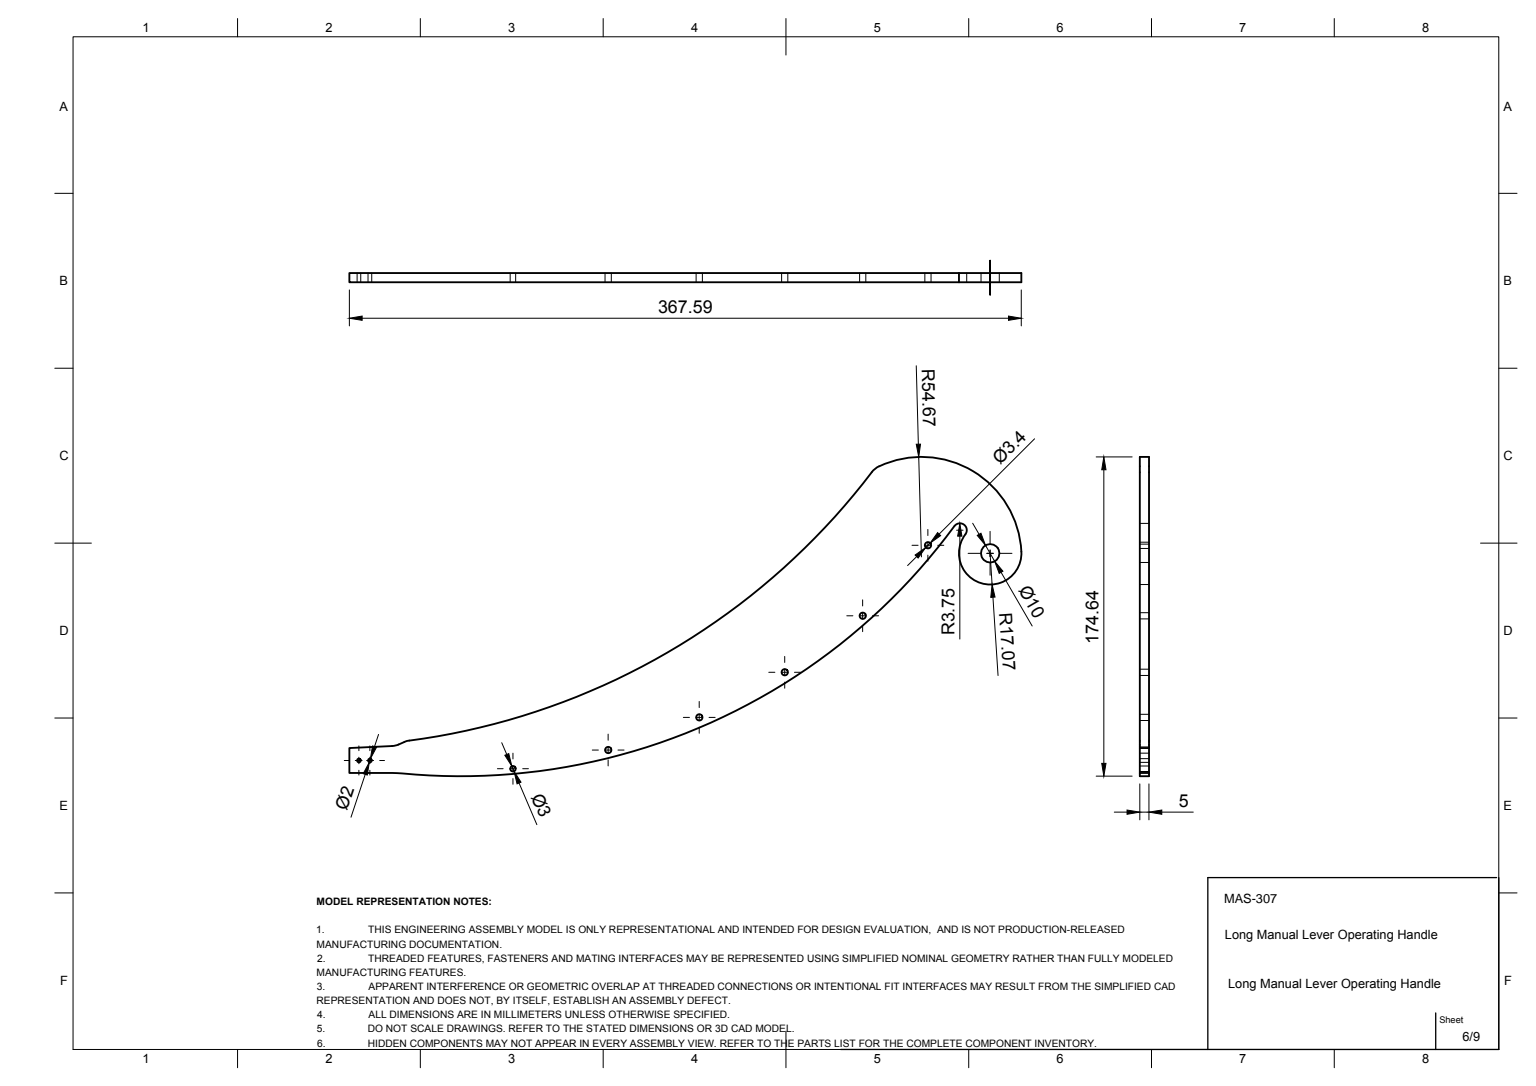
ISO-10303-21;
HEADER;
FILE_DESCRIPTION (('STEP AP214'),
    '1' );
FILE_NAME ('Long Manual Lever Operating Handle.step',
    '2026-10-06T07:34:29',
    ( '' ),
    ( '' ),
    'SwSTEP 2.0',
    'SolidWorks 2025',
    '' );
FILE_SCHEMA (( 'AUTOMOTIVE_DESIGN' ));
ENDSEC;

DATA;
#26=LINE ( 'NONE', #1296, #2230 ) ;
#32=ORIENTED_EDGE ( 'NONE', *, *, #11983, .F. ) ;
#34=DIRECTION ( 'NONE',  ( -0.000000000000000000, -0.000000000000000000, 1.000000000000000000 ) ) ;
#57=DIRECTION ( 'NONE',  ( 1.000000000000000000, 0.000000000000000000, 0.000000000000000000 ) ) ;
#79=ORIENTED_EDGE ( 'NONE', *, *, #3059, .T. ) ;
#100=DIRECTION ( 'NONE',  ( -1.000000000000000000, 0.000000000000000000, 0.000000000000000000 ) ) ;
#106=CYLINDRICAL_SURFACE ( 'NONE', #2526, 3.752352628381527833 ) ;
#107=LINE ( 'NONE', #4949, #8591 ) ;
#149=ORIENTED_EDGE ( 'NONE', *, *, #15360, .T. ) ;
#179=DIRECTION ( 'NONE',  ( 0.000000000000000000, 0.000000000000000000, 1.000000000000000000 ) ) ;
#192=ORIENTED_EDGE ( 'NONE', *, *, #11037, .F. ) ;
#214=VECTOR ( 'NONE', #12787, 1000.000000000000227 ) ;
#215=ORIENTED_EDGE ( 'NONE', *, *, #12661, .T. ) ;
#230=EDGE_LOOP ( 'NONE', ( #7966, #6489 ) ) ;
#255=DIRECTION ( 'NONE',  ( -0.000000000000000000, -0.000000000000000000, 1.000000000000000000 ) ) ;
#261=VECTOR ( 'NONE', #6975, 1000.000000000000000 ) ;
#284=CARTESIAN_POINT ( 'NONE',  ( 71.96535645333923981, 38.79159067395544014, 0.000000000000000000 ) ) ;
#289=AXIS2_PLACEMENT_3D ( 'NONE', #7420, #5036, #8676 ) ;
#295=VERTEX_POINT ( 'NONE', #2676 ) ;
#307=( NAMED_UNIT ( * ) SI_UNIT ( $, .STERADIAN. ) SOLID_ANGLE_UNIT ( ) );
#320=AXIS2_PLACEMENT_3D ( 'NONE', #10803, #2269, #8291 ) ;
#343=MECHANICAL_DESIGN_GEOMETRIC_PRESENTATION_REPRESENTATION('',(#14469),#13976);
#344=CARTESIAN_POINT ( 'NONE',  ( 70.26535645333922275, 38.79159067395544014, 5.000000000000000000 ) ) ;
#362=EDGE_CURVE ( 'NONE', #3997, #6369, #2486, .T. ) ;
#380=EDGE_CURVE ( 'NONE', #4418, #13651, #9757, .T. ) ;
#392=EDGE_CURVE ( 'NONE', #873, #13090, #3748, .T. ) ;
#401=EDGE_CURVE ( 'NONE', #462, #12631, #776, .T. ) ;
#437=CARTESIAN_POINT ( 'NONE',  ( -157.8787660911425803, 118.6941998492684149, 0.000000000000000000 ) ) ;
#462=VERTEX_POINT ( 'NONE', #13132 ) ;
#479=DIRECTION ( 'NONE',  ( 1.000000000000000000, 0.000000000000000000, 0.000000000000000000 ) ) ;
#518=EDGE_CURVE ( 'NONE', #13949, #12631, #4054, .T. ) ;
#523=AXIS2_PLACEMENT_3D ( 'NONE', #7628, #7709, #8968 ) ;
#535=ADVANCED_FACE ( 'NONE', ( #6521 ), #1971, .F. ) ;
#539=DIRECTION ( 'NONE',  ( 0.000000000000000000, 0.000000000000000000, 1.000000000000000000 ) ) ;
#545=CARTESIAN_POINT ( 'NONE',  ( -83.77455057502459113, 65.19100426474074084, 0.000000000000000000 ) ) ;
#548=DIRECTION ( 'NONE',  ( -1.000000000000000000, 0.000000000000000000, 0.000000000000000000 ) ) ;
#555=VERTEX_POINT ( 'NONE', #2885 ) ;
#565=VECTOR ( 'NONE', #10580, 1000.000000000000000 ) ;
#595=CARTESIAN_POINT ( 'NONE',  ( -164.5262273476079713, 106.7842295329138835, 5.000000000000000000 ) ) ;
#603=DIRECTION ( 'NONE',  ( 1.000000000000000000, 0.000000000000000000, 0.000000000000000000 ) ) ;
#617=LINE ( 'NONE', #4250, #8359 ) ;
#631=ORIENTED_EDGE ( 'NONE', *, *, #14587, .T. ) ;
#653=AXIS2_PLACEMENT_3D ( 'NONE', #7411, #179, #5028 ) ;
#667=ORIENTED_EDGE ( 'NONE', *, *, #9159, .T. ) ;
#673=CARTESIAN_POINT ( 'NONE',  ( -130.9946291778373961, 96.97121815129470690, 5.000000000000000000 ) ) ;
#678=AXIS2_PLACEMENT_3D ( 'NONE', #4721, #11915, #10972 ) ;
#679=FACE_BOUND ( 'NONE', #3096, .T. ) ;
#680=DIRECTION ( 'NONE',  ( 1.000000000000000000, 0.000000000000000000, 0.000000000000000000 ) ) ;
#681=EDGE_CURVE ( 'NONE', #5691, #12864, #13249, .T. ) ;
#697=ORIENTED_EDGE ( 'NONE', *, *, #1397, .T. ) ;
#751=CARTESIAN_POINT ( 'NONE',  ( 122.5806775638430253, 45.00321902537314145, 10.00000000000000178 ) ) ;
#760=CIRCLE ( 'NONE', #10878, 17.06579782980005433 ) ;
#768=CYLINDRICAL_SURFACE ( 'NONE', #9832, 1.699999999999993072 ) ;
#776=CIRCLE ( 'NONE', #15400, 5.000000000000004441 ) ;
#817=AXIS2_PLACEMENT_3D ( 'NONE', #1888, #15144, #9176 ) ;
#822=EDGE_CURVE ( 'NONE', #13988, #1469, #4075, .T. ) ;
#825=DIRECTION ( 'NONE',  ( -0.000000000000000000, -0.000000000000000000, -1.000000000000000000 ) ) ;
#839=EDGE_CURVE ( 'NONE', #6369, #8350, #8141, .T. ) ;
#844=FACE_BOUND ( 'NONE', #3836, .T. ) ;
#846=ORIENTED_EDGE ( 'NONE', *, *, #12928, .T. ) ;
#860=AXIS2_PLACEMENT_3D ( 'NONE', #12437, #4145, #5109 ) ;
#873=VERTEX_POINT ( 'NONE', #10108 ) ;
#876=CARTESIAN_POINT ( 'NONE',  ( 200.1062858801516597, 40.86394065090267702, 5.000000000000000000 ) ) ;
#895=EDGE_CURVE ( 'NONE', #11510, #13090, #8296, .T. ) ;
#902=DIRECTION ( 'NONE',  ( 0.000000000000000000, 0.000000000000000000, 1.000000000000000000 ) ) ;
#913=CARTESIAN_POINT ( 'NONE',  ( -150.4086188282879277, 107.2728346664360259, 0.000000000000000000 ) ) ;
#916=EDGE_CURVE ( 'NONE', #14981, #2732, #12150, .T. ) ;
#920=CYLINDRICAL_SURFACE ( 'NONE', #10681, 1.500000000000001332 ) ;
#955=ORIENTED_EDGE ( 'NONE', *, *, #7157, .T. ) ;
#963=ORIENTED_EDGE ( 'NONE', *, *, #5376, .T. ) ;
#970=CIRCLE ( 'NONE', #11577, 335.5619230110239641 ) ;
#1018=EDGE_LOOP ( 'NONE', ( #2531, #11475, #6093, #963 ) ) ;
#1037=CARTESIAN_POINT ( 'NONE',  ( -156.6477983077465410, 110.1970436846185066, -5.000000000000000000 ) ) ;
#1040=VECTOR ( 'NONE', #1882, 1000.000000000000227 ) ;
#1046=CARTESIAN_POINT ( 'NONE',  ( -135.3034657297974093, 107.4444500778096483, 5.000000000000000000 ) ) ;
#1059=ADVANCED_FACE ( 'NONE', ( #12139 ), #2593, .T. ) ;
#1071=VERTEX_POINT ( 'NONE', #6301 ) ;
#1092=DIRECTION ( 'NONE',  ( -0.000000000000000000, -0.000000000000000000, -1.000000000000000000 ) ) ;
#1121=DIRECTION ( 'NONE',  ( 1.000000000000000000, 0.000000000000000000, 0.000000000000000000 ) ) ;
#1126=VERTEX_POINT ( 'NONE', #4961 ) ;
#1152=DIRECTION ( 'NONE',  ( 1.000000000000000000, 0.000000000000000000, 0.000000000000000000 ) ) ;
#1153=DIRECTION ( 'NONE',  ( 0.000000000000000000, 0.000000000000000000, 1.000000000000000000 ) ) ;
#1163=EDGE_CURVE ( 'NONE', #4062, #3314, #3306, .T. ) ;
#1174=ORIENTED_EDGE ( 'NONE', *, *, #12928, .F. ) ;
#1197=ORIENTED_EDGE ( 'NONE', *, *, #13835, .T. ) ;
#1201=ADVANCED_FACE ( 'NONE', ( #14881 ), #9062, .F. ) ;
#1213=DIRECTION ( 'NONE',  ( 0.000000000000000000, 0.000000000000000000, 1.000000000000000000 ) ) ;
#1223=DIRECTION ( 'NONE',  ( 1.000000000000000000, 0.000000000000000000, 0.000000000000000000 ) ) ;
#1247=CIRCLE ( 'NONE', #3275, 1.000000000000000888 ) ;
#1252=AXIS2_PLACEMENT_3D ( 'NONE', #10138, #10216, #6512 ) ;
#1269=VERTEX_POINT ( 'NONE', #11422 ) ;
#1270=ORIENTED_EDGE ( 'NONE', *, *, #2769, .F. ) ;
#1296=CARTESIAN_POINT ( 'NONE',  ( -157.6477983077465694, 110.1970436846185066, -5.000000000000000000 ) ) ;
#1303=AXIS2_PLACEMENT_3D ( 'NONE', #9004, #12617, #1876 ) ;
#1312=FACE_OUTER_BOUND ( 'NONE', #2942, .T. ) ;
#1321=CYLINDRICAL_SURFACE ( 'NONE', #6253, 1.700000000000007061 ) ;
#1336=ORIENTED_EDGE ( 'NONE', *, *, #8208, .T. ) ;
#1388=EDGE_LOOP ( 'NONE', ( #7148, #8695 ) ) ;
#1397=EDGE_CURVE ( 'NONE', #14981, #13397, #2338, .T. ) ;
#1447=VERTEX_POINT ( 'NONE', #2261 ) ;
#1454=DIRECTION ( 'NONE',  ( 0.000000000000000000, 0.000000000000000000, 1.000000000000000000 ) ) ;
#1459=VECTOR ( 'NONE', #9027, 1000.000000000000000 ) ;
#1469=VERTEX_POINT ( 'NONE', #3451 ) ;
#1497=CIRCLE ( 'NONE', #10338, 9.999999999999994671 ) ;
#1508=EDGE_CURVE ( 'NONE', #11510, #12123, #1497, .T. ) ;
#1523=ADVANCED_FACE ( 'NONE', ( #15584 ), #7177, .F. ) ;
#1563=DIRECTION ( 'NONE',  ( -0.000000000000000000, -0.000000000000000000, 1.000000000000000000 ) ) ;
#1584=VERTEX_POINT ( 'NONE', #7772 ) ;
#1593=ORIENTED_EDGE ( 'NONE', *, *, #7358, .F. ) ;
#1598=DIRECTION ( 'NONE',  ( 0.9951762285753402715, -0.09810338464376282264, 0.000000000000000000 ) ) ;
#1625=EDGE_CURVE ( 'NONE', #11700, #462, #12561, .T. ) ;
#1644=EDGE_LOOP ( 'NONE', ( #4661, #10401 ) ) ;
#1648=ADVANCED_FACE ( 'NONE', ( #13749 ), #4122, .F. ) ;
#1674=CARTESIAN_POINT ( 'NONE',  ( 170.2911098586863545, 111.9959133412127272, 5.000000000000000000 ) ) ;
#1678=FACE_OUTER_BOUND ( 'NONE', #14769, .T. ) ;
#1681=CARTESIAN_POINT ( 'NONE',  ( -34.79899788034579444, 48.72489408690345414, 10.00000000000000178 ) ) ;
#1694=ADVANCED_FACE ( 'NONE', ( #1678 ), #5396, .T. ) ;
#1717=FACE_OUTER_BOUND ( 'NONE', #9914, .T. ) ;
#1742=CARTESIAN_POINT ( 'NONE',  ( 205.1062858801516597, 40.86394065090267702, 0.000000000000000000 ) ) ;
#1744=CARTESIAN_POINT ( 'NONE',  ( -144.0627431139473345, 95.36268816863731956, 5.000000000000000000 ) ) ;
#1753=EDGE_CURVE ( 'NONE', #1584, #14280, #107, .T. ) ;
#1756=CIRCLE ( 'NONE', #5285, 1.700000000000007061 ) ;
#1765=CARTESIAN_POINT ( 'NONE',  ( -133.4717610386620095, 107.2638826318553953, 0.000000000000000000 ) ) ;
#1776=DIRECTION ( 'NONE',  ( 0.000000000000000000, 0.000000000000000000, 1.000000000000000000 ) ) ;
#1785=VERTEX_POINT ( 'NONE', #3412 ) ;
#1799=AXIS2_PLACEMENT_3D ( 'NONE', #10657, #13006, #14345 ) ;
#1800=CARTESIAN_POINT ( 'NONE',  ( -133.4717610386620095, 107.2638826318553953, 5.000000000000000000 ) ) ;
#1835=DIRECTION ( 'NONE',  ( -0.000000000000000000, -0.000000000000000000, 1.000000000000000000 ) ) ;
#1839=DIRECTION ( 'NONE',  ( 0.4873681696970814103, 0.8731965799097685110, 0.000000000000000000 ) ) ;
#1876=DIRECTION ( 'NONE',  ( 1.000000000000000000, 0.000000000000000000, 0.000000000000000000 ) ) ;
#1877=ORIENTED_EDGE ( 'NONE', *, *, #5337, .T. ) ;
#1882=DIRECTION ( 'NONE',  ( -0.9951762285753402715, 0.09810338464376280876, -0.000000000000000000 ) ) ;
#1888=CARTESIAN_POINT ( 'NONE',  ( 122.5806775638430253, 45.00321902537314145, 0.000000000000000000 ) ) ;
#1895=FACE_OUTER_BOUND ( 'NONE', #5225, .T. ) ;
#1899=ADVANCED_FACE ( 'NONE', ( #14214 ), #11863, .F. ) ;
#1918=CARTESIAN_POINT ( 'NONE',  ( 70.26535645333922275, 38.79159067395544014, 0.000000000000000000 ) ) ;
#1923=FACE_BOUND ( 'NONE', #2485, .T. ) ;
#1971=CYLINDRICAL_SURFACE ( 'NONE', #523, 1.700000000000007061 ) ;
#1977=ORIENTED_EDGE ( 'NONE', *, *, #15100, .F. ) ;
#1992=DIRECTION ( 'NONE',  ( 1.000000000000000000, 0.000000000000000000, 0.000000000000000000 ) ) ;
#2009=AXIS2_PLACEMENT_3D ( 'NONE', #7353, #9634, #6085 ) ;
#2033=CARTESIAN_POINT ( 'NONE',  ( 70.26535645333922275, 38.79159067395544014, 5.000000000000000000 ) ) ;
#2034=CIRCLE ( 'NONE', #13636, 3.752352628381527833 ) ;
#2045=VECTOR ( 'NONE', #14822, 1000.000000000000000 ) ;
#2048=ORIENTED_EDGE ( 'NONE', *, *, #14989, .F. ) ;
#2052=ORIENTED_EDGE ( 'NONE', *, *, #10291, .T. ) ;
#2081=ORIENTED_EDGE ( 'NONE', *, *, #916, .T. ) ;
#2103=ORIENTED_EDGE ( 'NONE', *, *, #380, .F. ) ;
#2114=DIRECTION ( 'NONE',  ( -0.000000000000000000, -0.000000000000000000, -1.000000000000000000 ) ) ;
#2121=ORIENTED_EDGE ( 'NONE', *, *, #6897, .F. ) ;
#2122=CARTESIAN_POINT ( 'NONE',  ( 19.11029453487719110, 40.04259805664093363, 5.000000000000000000 ) ) ;
#2129=ORIENTED_EDGE ( 'NONE', *, *, #12783, .T. ) ;
#2132=CARTESIAN_POINT ( 'NONE',  ( -155.6477983077465410, 110.1970436846185066, -5.000000000000000000 ) ) ;
#2140=DIRECTION ( 'NONE',  ( -0.000000000000000000, -0.000000000000000000, -1.000000000000000000 ) ) ;
#2169=EDGE_CURVE ( 'NONE', #8061, #13697, #760, .T. ) ;
#2180=EDGE_LOOP ( 'NONE', ( #5222, #7079 ) ) ;
#2183=CARTESIAN_POINT ( 'NONE',  ( -85.27455057502459113, 65.19100426474074084, -20.00000000000000000 ) ) ;
#2191=DIRECTION ( 'NONE',  ( 1.000000000000000000, 0.000000000000000000, 0.000000000000000000 ) ) ;
#2207=EDGE_LOOP ( 'NONE', ( #7998, #697, #11706, #6584 ) ) ;
#2224=CIRCLE ( 'NONE', #4232, 1.500000000000001332 ) ;
#2230=VECTOR ( 'NONE', #255, 1000.000000000000000 ) ;
#2234=ORIENTED_EDGE ( 'NONE', *, *, #8634, .F. ) ;
#2261=CARTESIAN_POINT ( 'NONE',  ( -127.3091761562077409, 106.2673160437096413, 5.000000000000000000 ) ) ;
#2269=DIRECTION ( 'NONE',  ( -0.000000000000000000, -0.000000000000000000, 1.000000000000000000 ) ) ;
#2274=DIRECTION ( 'NONE',  ( 1.000000000000000000, 0.000000000000000000, 0.000000000000000000 ) ) ;
#2320=UNCERTAINTY_MEASURE_WITH_UNIT (LENGTH_MEASURE( 1.000000000000000082E-05 ), #15284, 'distance_accuracy_value', 'NONE');
#2338=LINE ( 'NONE', #3444, #2514 ) ;
#2356=EDGE_LOOP ( 'NONE', ( #9737, #192 ) ) ;
#2366=EDGE_CURVE ( 'NONE', #14692, #10673, #617, .T. ) ;
#2367=ORIENTED_EDGE ( 'NONE', *, *, #2169, .F. ) ;
#2375=VECTOR ( 'NONE', #1092, 1000.000000000000000 ) ;
#2377=ORIENTED_EDGE ( 'NONE', *, *, #9816, .F. ) ;
#2415=AXIS2_PLACEMENT_3D ( 'NONE', #9182, #9104, #548 ) ;
#2419=CARTESIAN_POINT ( 'NONE',  ( 174.2293059057019775, 61.25683321636181233, 5.000000000000000000 ) ) ;
#2457=EDGE_CURVE ( 'NONE', #9826, #13697, #3699, .T. ) ;
#2474=DIRECTION ( 'NONE',  ( 1.000000000000000000, 0.000000000000000000, -0.000000000000000000 ) ) ;
#2478=CARTESIAN_POINT ( 'NONE',  ( 51.07686401294030532, 368.7106150007013525, 0.000000000000000000 ) ) ;
#2485=EDGE_LOOP ( 'NONE', ( #149, #2081 ) ) ;
#2486=LINE ( 'NONE', #8430, #3319 ) ;
#2498=CIRCLE ( 'NONE', #6547, 9.999999999999994671 ) ;
#2499=CARTESIAN_POINT ( 'NONE',  ( 170.8293059057019718, 61.25683321636181233, 0.000000000000000000 ) ) ;
#2503=CYLINDRICAL_SURFACE ( 'NONE', #320, 1.700000000000000178 ) ;
#2505=AXIS2_PLACEMENT_3D ( 'NONE', #4185, #11387, #5471 ) ;
#2511=DIRECTION ( 'NONE',  ( 0.000000000000000000, 0.000000000000000000, 1.000000000000000000 ) ) ;
#2514=VECTOR ( 'NONE', #9523, 1000.000000000000000 ) ;
#2515=CARTESIAN_POINT ( 'NONE',  ( -33.09899788034579871, 48.72489408690345414, 5.000000000000000000 ) ) ;
#2526=AXIS2_PLACEMENT_3D ( 'NONE', #12047, #3605, #9766 ) ;
#2531=ORIENTED_EDGE ( 'NONE', *, *, #8498, .T. ) ;
#2533=VERTEX_POINT ( 'NONE', #9632 ) ;
#2542=AXIS2_PLACEMENT_3D ( 'NONE', #5724, #10700, #12740 ) ;
#2547=DIRECTION ( 'NONE',  ( -0.000000000000000000, -0.000000000000000000, 1.000000000000000000 ) ) ;
#2559=ORIENTED_EDGE ( 'NONE', *, *, #8634, .T. ) ;
#2593=CYLINDRICAL_SURFACE ( 'NONE', #289, 335.5619230110239641 ) ;
#2602=DIRECTION ( 'NONE',  ( 0.000000000000000000, 0.000000000000000000, 1.000000000000000000 ) ) ;
#2615=LINE ( 'NONE', #7439, #2045 ) ;
#2617=VERTEX_POINT ( 'NONE', #6553 ) ;
#2626=CIRCLE ( 'NONE', #9687, 1.500000000000001332 ) ;
#2640=DIRECTION ( 'NONE',  ( 0.000000000000000000, 0.000000000000000000, 1.000000000000000000 ) ) ;
#2654=VERTEX_POINT ( 'NONE', #12524 ) ;
#2666=AXIS2_PLACEMENT_3D ( 'NONE', #12786, #5543, #3098 ) ;
#2676=CARTESIAN_POINT ( 'NONE',  ( 68.56535645333921991, 38.79159067395544014, 5.000000000000000000 ) ) ;
#2681=AXIS2_PLACEMENT_3D ( 'NONE', #673, #11677, #3216 ) ;
#2705=ORIENTED_EDGE ( 'NONE', *, *, #13825, .T. ) ;
#2732=VERTEX_POINT ( 'NONE', #913 ) ;
#2733=VECTOR ( 'NONE', #9153, 1000.000000000000000 ) ;
#2752=LINE ( 'NONE', #11200, #9169 ) ;
#2769=EDGE_CURVE ( 'NONE', #2533, #9826, #15516, .T. ) ;
#2770=EDGE_CURVE ( 'NONE', #13816, #5538, #14017, .T. ) ;
#2790=EDGE_LOOP ( 'NONE', ( #5117, #15465 ) ) ;
#2794=AXIS2_PLACEMENT_3D ( 'NONE', #9407, #2511, #6227 ) ;
#2800=FACE_OUTER_BOUND ( 'NONE', #1018, .T. ) ;
#2826=CARTESIAN_POINT ( 'NONE',  ( 215.4200305399390345, 33.33196348269225240, 0.000000000000000000 ) ) ;
#2870=ORIENTED_EDGE ( 'NONE', *, *, #1625, .F. ) ;
#2885=CARTESIAN_POINT ( 'NONE',  ( 170.8293059057019718, 61.25683321636181233, 5.000000000000000000 ) ) ;
#2887=CIRCLE ( 'NONE', #9443, 54.67486482576605766 ) ;
#2938=EDGE_CURVE ( 'NONE', #1447, #1126, #13504, .T. ) ;
#2942=EDGE_LOOP ( 'NONE', ( #2870, #2121, #10598, #12745 ) ) ;
#2944=AXIS2_PLACEMENT_3D ( 'NONE', #6456, #5104, #11261 ) ;
#2946=ORIENTED_EDGE ( 'NONE', *, *, #9969, .F. ) ;
#2967=EDGE_CURVE ( 'NONE', #12864, #2654, #10754, .T. ) ;
#2969=CARTESIAN_POINT ( 'NONE',  ( 17.41029453487719181, 40.04259805664093363, 5.000000000000000000 ) ) ;
#2999=ORIENTED_EDGE ( 'NONE', *, *, #3303, .T. ) ;
#3011=ORIENTED_EDGE ( 'NONE', *, *, #362, .T. ) ;
#3019=CIRCLE ( 'NONE', #13582, 335.5619230110239641 ) ;
#3059=EDGE_CURVE ( 'NONE', #3997, #6520, #9751, .T. ) ;
#3065=ORIENTED_EDGE ( 'NONE', *, *, #9925, .F. ) ;
#3089=EDGE_CURVE ( 'NONE', #5874, #4096, #3447, .T. ) ;
#3090=FACE_OUTER_BOUND ( 'NONE', #2207, .T. ) ;
#3092=PRODUCT_CONTEXT ( 'NONE', #15303, 'mechanical' ) ;
#3096=EDGE_LOOP ( 'NONE', ( #10306, #7313 ) ) ;
#3098=DIRECTION ( 'NONE',  ( 1.000000000000000000, 0.000000000000000000, 0.000000000000000000 ) ) ;
#3102=CARTESIAN_POINT ( 'NONE',  ( -36.49899788034579018, 48.72489408690345414, 0.000000000000000000 ) ) ;
#3146=CARTESIAN_POINT ( 'NONE',  ( -150.4086188282879277, 107.2728346664360259, 5.000000000000000000 ) ) ;
#3152=DIRECTION ( 'NONE',  ( 0.000000000000000000, 0.000000000000000000, -1.000000000000000000 ) ) ;
#3160=CIRCLE ( 'NONE', #5179, 1.700000000000000178 ) ;
#3161=CYLINDRICAL_SURFACE ( 'NONE', #15186, 1.000000000000000888 ) ;
#3185=ORIENTED_EDGE ( 'NONE', *, *, #4300, .T. ) ;
#3216=DIRECTION ( 'NONE',  ( -1.000000000000000000, 0.000000000000000000, 0.000000000000000000 ) ) ;
#3230=LINE ( 'NONE', #14119, #2375 ) ;
#3240=ADVANCED_FACE ( 'NONE', ( #14079 ), #6919, .F. ) ;
#3245=VERTEX_POINT ( 'NONE', #7235 ) ;
#3247=ORIENTED_EDGE ( 'NONE', *, *, #1753, .T. ) ;
#3259=VECTOR ( 'NONE', #4688, 1000.000000000000000 ) ;
#3263=VERTEX_POINT ( 'NONE', #5881 ) ;
#3264=CARTESIAN_POINT ( 'NONE',  ( 172.5293059057019889, 61.25683321636181233, 10.00000000000000178 ) ) ;
#3275=AXIS2_PLACEMENT_3D ( 'NONE', #13025, #14216, #6677 ) ;
#3282=AXIS2_PLACEMENT_3D ( 'NONE', #3576, #4757, #12965 ) ;
#3289=DIRECTION ( 'NONE',  ( -1.000000000000000000, 0.000000000000000000, 0.000000000000000000 ) ) ;
#3303=EDGE_CURVE ( 'NONE', #11700, #13949, #9738, .T. ) ;
#3304=DIRECTION ( 'NONE',  ( -0.000000000000000000, -0.000000000000000000, 1.000000000000000000 ) ) ;
#3306=CIRCLE ( 'NONE', #12125, 1.699999999999993072 ) ;
#3307=DIRECTION ( 'NONE',  ( 0.000000000000000000, 0.000000000000000000, 1.000000000000000000 ) ) ;
#3314=VERTEX_POINT ( 'NONE', #10620 ) ;
#3319=VECTOR ( 'NONE', #6126, 1000.000000000000000 ) ;
#3339=DIRECTION ( 'NONE',  ( -1.000000000000000000, 0.000000000000000000, 0.000000000000000000 ) ) ;
#3364=AXIS2_PLACEMENT_3D ( 'NONE', #3610, #10802, #9534 ) ;
#3366=CARTESIAN_POINT ( 'NONE',  ( 165.1224552381025887, 111.1124422548786299, 5.000000000000000000 ) ) ;
#3377=CIRCLE ( 'NONE', #15457, 1.700000000000007061 ) ;
#3382=FACE_OUTER_BOUND ( 'NONE', #12254, .T. ) ;
#3409=LINE ( 'NONE', #13021, #261 ) ;
#3410=AXIS2_PLACEMENT_3D ( 'NONE', #14547, #8891, #12496 ) ;
#3412=CARTESIAN_POINT ( 'NONE',  ( 120.8806775638430224, 45.00321902537314145, 5.000000000000000000 ) ) ;
#3415=CIRCLE ( 'NONE', #2666, 1.699999999999993072 ) ;
#3435=CARTESIAN_POINT ( 'NONE',  ( -36.49899788034579018, 48.72489408690345414, 5.000000000000000000 ) ) ;
#3444=CARTESIAN_POINT ( 'NONE',  ( -152.4086188282879277, 107.2728346664360259, -5.000000000000000000 ) ) ;
#3447=CIRCLE ( 'NONE', #653, 1.700000000000007061 ) ;
#3451=CARTESIAN_POINT ( 'NONE',  ( -86.77455057502459113, 65.19100426474074084, 0.000000000000000000 ) ) ;
#3456=CARTESIAN_POINT ( 'NONE',  ( -152.4086188282879277, 107.2728346664360259, 5.000000000000000000 ) ) ;
#3463=ORIENTED_EDGE ( 'NONE', *, *, #9811, .F. ) ;
#3495=AXIS2_PLACEMENT_3D ( 'NONE', #1918, #13843, #6446 ) ;
#3497=CARTESIAN_POINT ( 'NONE',  ( 170.8293059057019718, 61.25683321636181233, 10.00000000000000178 ) ) ;
#3503=FACE_BOUND ( 'NONE', #13506, .T. ) ;
#3511=DIRECTION ( 'NONE',  ( 0.000000000000000000, 0.000000000000000000, 1.000000000000000000 ) ) ;
#3525=ADVANCED_FACE ( 'NONE', ( #2800 ), #6198, .F. ) ;
#3531=VECTOR ( 'NONE', #1563, 1000.000000000000000 ) ;
#3575=DIRECTION ( 'NONE',  ( 0.000000000000000000, 0.000000000000000000, 1.000000000000000000 ) ) ;
#3576=CARTESIAN_POINT ( 'NONE',  ( 13.07968152355895874, 460.3807876674321165, 5.000000000000000000 ) ) ;
#3578=DIRECTION ( 'NONE',  ( 0.000000000000000000, 0.000000000000000000, 1.000000000000000000 ) ) ;
#3589=DIRECTION ( 'NONE',  ( -1.000000000000000000, 0.000000000000000000, 0.000000000000000000 ) ) ;
#3603=ORIENTED_EDGE ( 'NONE', *, *, #7385, .T. ) ;
#3605=DIRECTION ( 'NONE',  ( -0.000000000000000000, -0.000000000000000000, -1.000000000000000000 ) ) ;
#3610=CARTESIAN_POINT ( 'NONE',  ( -151.4086188282879277, 107.2728346664360259, -5.000000000000000000 ) ) ;
#3699=LINE ( 'NONE', #13084, #5721 ) ;
#3719=ORIENTED_EDGE ( 'NONE', *, *, #14625, .F. ) ;
#3724=( NAMED_UNIT ( * ) PLANE_ANGLE_UNIT ( ) SI_UNIT ( $, .RADIAN. ) );
#3748=LINE ( 'NONE', #3833, #12138 ) ;
#3758=CIRCLE ( 'NONE', #9790, 1.700000000000000178 ) ;
#3768=DIRECTION ( 'NONE',  ( 1.000000000000000000, 0.000000000000000000, 0.000000000000000000 ) ) ;
#3769=CIRCLE ( 'NONE', #14339, 5.000000000000004441 ) ;
#3810=FILL_AREA_STYLE ('',( #12321 ) ) ;
#3825=EDGE_CURVE ( 'NONE', #13113, #15168, #5230, .T. ) ;
#3827=CIRCLE ( 'NONE', #12885, 380.9270036976043343 ) ;
#3833=CARTESIAN_POINT ( 'NONE',  ( -157.8787660911425803, 118.6941998492684149, 5.000000000000000000 ) ) ;
#3836=EDGE_LOOP ( 'NONE', ( #12094, #10696 ) ) ;
#3847=CARTESIAN_POINT ( 'NONE',  ( -156.6477983077465410, 110.1970436846185066, 5.000000000000000000 ) ) ;
#3851=FACE_OUTER_BOUND ( 'NONE', #5147, .T. ) ;
#3870=ORIENTED_EDGE ( 'NONE', *, *, #8268, .F. ) ;
#3873=EDGE_LOOP ( 'NONE', ( #11108, #14364, #10374, #5700 ) ) ;
#3917=ADVANCED_FACE ( 'NONE', ( #4426 ), #6670, .T. ) ;
#3925=ORIENTED_EDGE ( 'NONE', *, *, #10114, .T. ) ;
#3948=DIRECTION ( 'NONE',  ( 1.000000000000000000, 0.000000000000000000, 0.000000000000000000 ) ) ;
#3957=EDGE_LOOP ( 'NONE', ( #7121, #9893, #6894, #14139 ) ) ;
#3968=CYLINDRICAL_SURFACE ( 'NONE', #14362, 1.699999999999993072 ) ;
#3975=DIRECTION ( 'NONE',  ( 1.000000000000000000, 0.000000000000000000, 0.000000000000000000 ) ) ;
#3996=CIRCLE ( 'NONE', #12819, 17.06579782980005433 ) ;
#3997=VERTEX_POINT ( 'NONE', #15307 ) ;
#4014=ORIENTED_EDGE ( 'NONE', *, *, #2769, .T. ) ;
#4037=DIRECTION ( 'NONE',  ( 0.000000000000000000, 0.000000000000000000, 1.000000000000000000 ) ) ;
#4054=LINE ( 'NONE', #11248, #14897 ) ;
#4062=VERTEX_POINT ( 'NONE', #3102 ) ;
#4068=EDGE_CURVE ( 'NONE', #4062, #10761, #6814, .T. ) ;
#4075=CIRCLE ( 'NONE', #11906, 1.500000000000001332 ) ;
#4081=ORIENTED_EDGE ( 'NONE', *, *, #15451, .T. ) ;
#4096=VERTEX_POINT ( 'NONE', #13332 ) ;
#4114=CARTESIAN_POINT ( 'NONE',  ( 205.1062858801516597, 40.86394065090267702, 5.000000000000000000 ) ) ;
#4122=PLANE ( 'NONE',  #14857 ) ;
#4137=ORIENTED_EDGE ( 'NONE', *, *, #2366, .F. ) ;
#4139=DIRECTION ( 'NONE',  ( -0.000000000000000000, -0.000000000000000000, 1.000000000000000000 ) ) ;
#4145=DIRECTION ( 'NONE',  ( 0.000000000000000000, 0.000000000000000000, 1.000000000000000000 ) ) ;
#4151=CIRCLE ( 'NONE', #3410, 9.999999999999994671 ) ;
#4161=DIRECTION ( 'NONE',  ( -0.4873681696970814103, -0.8731965799097685110, -0.000000000000000000 ) ) ;
#4175=DIRECTION ( 'NONE',  ( -1.000000000000000000, 0.000000000000000000, 0.000000000000000000 ) ) ;
#4185=CARTESIAN_POINT ( 'NONE',  ( -151.4086188282879277, 107.2728346664360259, 0.000000000000000000 ) ) ;
#4204=CARTESIAN_POINT ( 'NONE',  ( -164.5262273476079713, 106.7842295329138835, 5.000000000000000000 ) ) ;
#4206=CARTESIAN_POINT ( 'NONE',  ( -152.4086188282879277, 107.2728346664360259, 0.000000000000000000 ) ) ;
#4210=ORIENTED_EDGE ( 'NONE', *, *, #392, .F. ) ;
#4232=AXIS2_PLACEMENT_3D ( 'NONE', #4459, #14168, #8038 ) ;
#4248=ORIENTED_EDGE ( 'NONE', *, *, #7157, .F. ) ;
#4250=CARTESIAN_POINT ( 'NONE',  ( 165.1224552381025887, 111.1124422548786299, 5.000000000000000000 ) ) ;
#4252=CIRCLE ( 'NONE', #11330, 1.699999999999993072 ) ;
#4261=LINE ( 'NONE', #1744, #10230 ) ;
#4277=EDGE_CURVE ( 'NONE', #6520, #2617, #970, .T. ) ;
#4298=ORIENTED_EDGE ( 'NONE', *, *, #7802, .T. ) ;
#4300=EDGE_CURVE ( 'NONE', #14293, #11510, #6722, .T. ) ;
#4324=DIRECTION ( 'NONE',  ( 1.000000000000000000, 0.000000000000000000, -0.000000000000000000 ) ) ;
#4340=EDGE_CURVE ( 'NONE', #4096, #8585, #10499, .T. ) ;
#4381=VERTEX_POINT ( 'NONE', #2122 ) ;
#4418=VERTEX_POINT ( 'NONE', #4644 ) ;
#4426=FACE_OUTER_BOUND ( 'NONE', #10145, .T. ) ;
#4459=CARTESIAN_POINT ( 'NONE',  ( -85.27455057502459113, 65.19100426474074084, 5.000000000000000000 ) ) ;
#4474=ADVANCED_FACE ( 'NONE', ( #8300 ), #1321, .F. ) ;
#4475=DIRECTION ( 'NONE',  ( 0.000000000000000000, 0.000000000000000000, 1.000000000000000000 ) ) ;
#4477=PLANE ( 'NONE',  #7844 ) ;
#4479=ORIENTED_EDGE ( 'NONE', *, *, #681, .F. ) ;
#4483=ORIENTED_EDGE ( 'NONE', *, *, #9364, .T. ) ;
#4500=ADVANCED_FACE ( 'NONE', ( #13080 ), #11837, .F. ) ;
#4515=VECTOR ( 'NONE', #13505, 1000.000000000000000 ) ;
#4520=DIRECTION ( 'NONE',  ( 1.000000000000000000, 0.000000000000000000, 0.000000000000000000 ) ) ;
#4523=AXIS2_PLACEMENT_3D ( 'NONE', #13781, #6544, #11343 ) ;
#4524=VERTEX_POINT ( 'NONE', #10731 ) ;
#4565=CARTESIAN_POINT ( 'NONE',  ( -151.4086188282879277, 107.2728346664360259, 0.000000000000000000 ) ) ;
#4568=CARTESIAN_POINT ( 'NONE',  ( 0.000000000000000000, 0.000000000000000000, 0.000000000000000000 ) ) ;
#4589=CARTESIAN_POINT ( 'NONE',  ( -34.79899788034579444, 48.72489408690345414, 5.000000000000000000 ) ) ;
#4595=EDGE_CURVE ( 'NONE', #4418, #1071, #3758, .T. ) ;
#4605=VERTEX_POINT ( 'NONE', #2515 ) ;
#4610=CARTESIAN_POINT ( 'NONE',  ( 124.2806775638430281, 45.00321902537314145, 5.000000000000000000 ) ) ;
#4633=AXIS2_PLACEMENT_3D ( 'NONE', #9385, #12997, #2191 ) ;
#4644=CARTESIAN_POINT ( 'NONE',  ( 15.71029453487719074, 40.04259805664093363, 0.000000000000000000 ) ) ;
#4650=ORIENTED_EDGE ( 'NONE', *, *, #10741, .T. ) ;
#4661=ORIENTED_EDGE ( 'NONE', *, *, #15012, .T. ) ;
#4663=CARTESIAN_POINT ( 'NONE',  ( -133.4717610386620095, 107.2638826318553953, 5.000000000000000000 ) ) ;
#4670=VECTOR ( 'NONE', #5871, 1000.000000000000227 ) ;
#4688=DIRECTION ( 'NONE',  ( -0.000000000000000000, -0.000000000000000000, 1.000000000000000000 ) ) ;
#4714=CARTESIAN_POINT ( 'NONE',  ( 13.07968152355895874, 460.3807876674321165, 5.000000000000000000 ) ) ;
#4721=CARTESIAN_POINT ( 'NONE',  ( 122.5806775638430253, 45.00321902537314145, 10.00000000000000178 ) ) ;
#4734=DIRECTION ( 'NONE',  ( -0.000000000000000000, -0.000000000000000000, 1.000000000000000000 ) ) ;
#4739=ORIENTED_EDGE ( 'NONE', *, *, #9954, .T. ) ;
#4755=CYLINDRICAL_SURFACE ( 'NONE', #12975, 5.000000000000004441 ) ;
#4757=DIRECTION ( 'NONE',  ( -0.000000000000000000, -0.000000000000000000, -1.000000000000000000 ) ) ;
#4764=DIRECTION ( 'NONE',  ( 0.000000000000000000, 0.000000000000000000, 1.000000000000000000 ) ) ;
#4768=LINE ( 'NONE', #13200, #3259 ) ;
#4790=AXIS2_PLACEMENT_3D ( 'NONE', #2183, #8282, #14174 ) ;
#4799=CARTESIAN_POINT ( 'NONE',  ( 68.56535645333921991, 38.79159067395544014, 0.000000000000000000 ) ) ;
#4805=CIRCLE ( 'NONE', #10363, 1.700000000000007061 ) ;
#4851=EDGE_CURVE ( 'NONE', #2533, #8061, #15199, .T. ) ;
#4858=EDGE_CURVE ( 'NONE', #4524, #6229, #12678, .T. ) ;
#4919=( LENGTH_UNIT ( ) NAMED_UNIT ( * ) SI_UNIT ( .MILLI., .METRE. ) );
#4930=FACE_BOUND ( 'NONE', #15283, .T. ) ;
#4931=DIRECTION ( 'NONE',  ( -1.000000000000000000, 0.000000000000000000, 0.000000000000000000 ) ) ;
#4936=ORIENTED_EDGE ( 'NONE', *, *, #2938, .F. ) ;
#4947=VERTEX_POINT ( 'NONE', #595 ) ;
#4949=CARTESIAN_POINT ( 'NONE',  ( 215.4200305399390345, 33.33196348269225240, 5.000000000000000000 ) ) ;
#4954=LINE ( 'NONE', #9772, #7670 ) ;
#4961=CARTESIAN_POINT ( 'NONE',  ( -130.0135953313997561, 106.9229804370480537, 5.000000000000000000 ) ) ;
#4993=DIRECTION ( 'NONE',  ( 1.000000000000000000, 0.000000000000000000, 0.000000000000000000 ) ) ;
#4998=CARTESIAN_POINT ( 'NONE',  ( 190.2479883433758800, 63.36949047362622167, 5.000000000000000000 ) ) ;
#5023=ORIENTED_EDGE ( 'NONE', *, *, #15012, .F. ) ;
#5028=DIRECTION ( 'NONE',  ( 1.000000000000000000, 0.000000000000000000, 0.000000000000000000 ) ) ;
#5036=DIRECTION ( 'NONE',  ( -0.000000000000000000, -0.000000000000000000, -1.000000000000000000 ) ) ;
#5104=DIRECTION ( 'NONE',  ( -0.000000000000000000, -0.000000000000000000, -1.000000000000000000 ) ) ;
#5109=DIRECTION ( 'NONE',  ( 1.000000000000000000, 0.000000000000000000, 0.000000000000000000 ) ) ;
#5117=ORIENTED_EDGE ( 'NONE', *, *, #9159, .F. ) ;
#5147=EDGE_LOOP ( 'NONE', ( #10082, #3185, #6835, #4210 ) ) ;
#5179=AXIS2_PLACEMENT_3D ( 'NONE', #12020, #3575, #1121 ) ;
#5183=DIRECTION ( 'NONE',  ( 1.000000000000000000, 0.000000000000000000, 0.000000000000000000 ) ) ;
#5194=EDGE_LOOP ( 'NONE', ( #2103, #14481, #846, #7845 ) ) ;
#5205=CARTESIAN_POINT ( 'NONE',  ( -164.5262273476079713, 106.7842295329138835, 0.000000000000000000 ) ) ;
#5222=ORIENTED_EDGE ( 'NONE', *, *, #6856, .T. ) ;
#5225=EDGE_LOOP ( 'NONE', ( #9851, #3463, #7929, #3011 ) ) ;
#5230=LINE ( 'NONE', #1674, #1459 ) ;
#5277=ORIENTED_EDGE ( 'NONE', *, *, #8268, .T. ) ;
#5285=AXIS2_PLACEMENT_3D ( 'NONE', #5560, #9120, #479 ) ;
#5297=AXIS2_PLACEMENT_3D ( 'NONE', #751, #34, #1223 ) ;
#5337=EDGE_CURVE ( 'NONE', #5538, #14046, #7114, .T. ) ;
#5348=ORIENTED_EDGE ( 'NONE', *, *, #14711, .T. ) ;
#5351=CARTESIAN_POINT ( 'NONE',  ( 124.2806775638430281, 45.00321902537314145, 10.00000000000000178 ) ) ;
#5376=EDGE_CURVE ( 'NONE', #4947, #7984, #3230, .T. ) ;
#5396=CYLINDRICAL_SURFACE ( 'NONE', #1252, 54.67486482576605766 ) ;
#5427=ORIENTED_EDGE ( 'NONE', *, *, #13085, .F. ) ;
#5437=CARTESIAN_POINT ( 'NONE',  ( 169.5018791832601721, 101.0521538385604003, 0.000000000000000000 ) ) ;
#5458=CARTESIAN_POINT ( 'NONE',  ( -151.4086188282879277, 107.2728346664360259, -5.000000000000000000 ) ) ;
#5467=ORIENTED_EDGE ( 'NONE', *, *, #4300, .F. ) ;
#5471=DIRECTION ( 'NONE',  ( 1.000000000000000000, 0.000000000000000000, 0.000000000000000000 ) ) ;
#5488=CARTESIAN_POINT ( 'NONE',  ( -151.4086188282879277, 107.2728346664360259, 5.000000000000000000 ) ) ;
#5510=DIRECTION ( 'NONE',  ( 0.8731965799097686221, -0.4873681696970812438, -0.000000000000000000 ) ) ;
#5516=CYLINDRICAL_SURFACE ( 'NONE', #2681, 10.00000000000000888 ) ;
#5523=FACE_BOUND ( 'NONE', #11626, .T. ) ;
#5535=CIRCLE ( 'NONE', #7558, 1.000000000000000888 ) ;
#5538=VERTEX_POINT ( 'NONE', #284 ) ;
#5543=DIRECTION ( 'NONE',  ( 0.000000000000000000, 0.000000000000000000, 1.000000000000000000 ) ) ;
#5560=CARTESIAN_POINT ( 'NONE',  ( 122.5806775638430253, 45.00321902537314145, 0.000000000000000000 ) ) ;
#5588=VECTOR ( 'NONE', #5929, 1000.000000000000000 ) ;
#5623=LINE ( 'NONE', #13982, #214 ) ;
#5628=ORIENTED_EDGE ( 'NONE', *, *, #15451, .F. ) ;
#5640=CARTESIAN_POINT ( 'NONE',  ( 200.1062858801516597, 40.86394065090267702, 5.000000000000000000 ) ) ;
#5656=CARTESIAN_POINT ( 'NONE',  ( 195.1062858801516597, 40.86394065090267702, 0.000000000000000000 ) ) ;
#5659=DIRECTION ( 'NONE',  ( 1.000000000000000000, -1.942890293094024892E-14, 0.000000000000000000 ) ) ;
#5681=DIRECTION ( 'NONE',  ( 1.000000000000000000, 0.000000000000000000, 0.000000000000000000 ) ) ;
#5691=VERTEX_POINT ( 'NONE', #9381 ) ;
#5700=ORIENTED_EDGE ( 'NONE', *, *, #1753, .F. ) ;
#5704=DIRECTION ( 'NONE',  ( 1.000000000000000000, 0.000000000000000000, 0.000000000000000000 ) ) ;
#5709=CARTESIAN_POINT ( 'NONE',  ( 200.1062858801516597, 40.86394065090267702, 5.000000000000000000 ) ) ;
#5721=VECTOR ( 'NONE', #11998, 1000.000000000000000 ) ;
#5724=CARTESIAN_POINT ( 'NONE',  ( -132.4907271922243694, 117.2156449176087847, 5.000000000000000000 ) ) ;
#5725=ORIENTED_EDGE ( 'NONE', *, *, #518, .F. ) ;
#5736=CARTESIAN_POINT ( 'NONE',  ( 172.5293059057019889, 61.25683321636181233, 5.000000000000000000 ) ) ;
#5765=EDGE_LOOP ( 'NONE', ( #3870, #14905, #11264, #9822 ) ) ;
#5779=FACE_OUTER_BOUND ( 'NONE', #3873, .T. ) ;
#5795=ORIENTED_EDGE ( 'NONE', *, *, #1508, .T. ) ;
#5805=VECTOR ( 'NONE', #1776, 1000.000000000000000 ) ;
#5871=DIRECTION ( 'NONE',  ( -0.9951762285753402715, 0.09810338464376280876, -0.000000000000000000 ) ) ;
#5873=CARTESIAN_POINT ( 'NONE',  ( -151.4086188282879277, 107.2728346664360259, 5.000000000000000000 ) ) ;
#5874=VERTEX_POINT ( 'NONE', #2499 ) ;
#5881=CARTESIAN_POINT ( 'NONE',  ( -127.3091761562077409, 106.2673160437096413, 0.000000000000000000 ) ) ;
#5929=DIRECTION ( 'NONE',  ( -0.000000000000000000, -0.000000000000000000, 1.000000000000000000 ) ) ;
#5942=AXIS2_PLACEMENT_3D ( 'NONE', #11727, #4139, #8979 ) ;
#5987=EDGE_CURVE ( 'NONE', #7301, #6998, #2626, .T. ) ;
#6002=AXIS2_PLACEMENT_3D ( 'NONE', #4714, #9309, #13071 ) ;
#6024=PRODUCT_DEFINITION_FORMATION_WITH_SPECIFIED_SOURCE ( 'ANY', '', #13944, .NOT_KNOWN. ) ;
#6031=EDGE_LOOP ( 'NONE', ( #5628, #5277, #631, #7140 ) ) ;
#6042=CARTESIAN_POINT ( 'NONE',  ( 166.3583383998781358, 57.46267437295986014, 5.000000000000000000 ) ) ;
#6048=AXIS2_PLACEMENT_3D ( 'NONE', #13027, #14147, #9500 ) ;
#6070=FACE_OUTER_BOUND ( 'NONE', #10551, .T. ) ;
#6085=DIRECTION ( 'NONE',  ( 1.000000000000000000, 0.000000000000000000, 0.000000000000000000 ) ) ;
#6093=ORIENTED_EDGE ( 'NONE', *, *, #12661, .F. ) ;
#6120=EDGE_CURVE ( 'NONE', #4381, #13651, #8688, .T. ) ;
#6126=DIRECTION ( 'NONE',  ( -0.000000000000000000, -0.000000000000000000, -1.000000000000000000 ) ) ;
#6191=CARTESIAN_POINT ( 'NONE',  ( -34.79899788034579444, 48.72489408690345414, 0.000000000000000000 ) ) ;
#6197=FACE_OUTER_BOUND ( 'NONE', #6875, .T. ) ;
#6198=PLANE ( 'NONE',  #8723 ) ;
#6226=ORIENTED_EDGE ( 'NONE', *, *, #4068, .T. ) ;
#6227=DIRECTION ( 'NONE',  ( 1.000000000000000000, 0.000000000000000000, 0.000000000000000000 ) ) ;
#6229=VERTEX_POINT ( 'NONE', #4610 ) ;
#6241=EDGE_LOOP ( 'NONE', ( #13369, #1197, #10050, #7708 ) ) ;
#6253=AXIS2_PLACEMENT_3D ( 'NONE', #14269, #10656, #7111 ) ;
#6268=( GEOMETRIC_REPRESENTATION_CONTEXT ( 3 ) GLOBAL_UNCERTAINTY_ASSIGNED_CONTEXT ( ( #2320 ) ) GLOBAL_UNIT_ASSIGNED_CONTEXT ( ( #15284, #13078, #11913 ) ) REPRESENTATION_CONTEXT ( 'NONE', 'WORKASPACE' ) );
#6272=CARTESIAN_POINT ( 'NONE',  ( -139.4318739252458670, 92.47118091487817537, 5.000000000000000000 ) ) ;
#6276=AXIS2_PLACEMENT_3D ( 'NONE', #5488, #7945, #3975 ) ;
#6301=CARTESIAN_POINT ( 'NONE',  ( 19.11029453487719110, 40.04259805664093363, 0.000000000000000000 ) ) ;
#6308=CARTESIAN_POINT ( 'NONE',  ( -139.4318739252458670, 92.47118091487817537, 0.000000000000000000 ) ) ;
#6320=ADVANCED_FACE ( 'NONE', ( #12737, #1923, #15178, #3503, #9510, #8494, #13276, #4930, #8341, #6197 ), #12104, .F. ) ;
#6321=CARTESIAN_POINT ( 'NONE',  ( 170.2911098586863545, 111.9959133412127272, 5.000000000000000000 ) ) ;
#6364=ORIENTED_EDGE ( 'NONE', *, *, #3825, .F. ) ;
#6369=VERTEX_POINT ( 'NONE', #12030 ) ;
#6373=ORIENTED_EDGE ( 'NONE', *, *, #2457, .F. ) ;
#6398=CIRCLE ( 'NONE', #817, 1.700000000000007061 ) ;
#6410=DIRECTION ( 'NONE',  ( -1.000000000000000000, 0.000000000000000000, 0.000000000000000000 ) ) ;
#6442=EDGE_LOOP ( 'NONE', ( #12175, #14003 ) ) ;
#6446=DIRECTION ( 'NONE',  ( 1.000000000000000000, 0.000000000000000000, 0.000000000000000000 ) ) ;
#6454=AXIS2_PLACEMENT_3D ( 'NONE', #3264, #10147, #13996 ) ;
#6456=CARTESIAN_POINT ( 'NONE',  ( -173.4445345933175986, 43.15250799526725700, 5.000000000000000000 ) ) ;
#6483=CARTESIAN_POINT ( 'NONE',  ( 183.0404880503516267, 40.86394065090267702, 0.000000000000000000 ) ) ;
#6489=ORIENTED_EDGE ( 'NONE', *, *, #3089, .T. ) ;
#6495=CARTESIAN_POINT ( 'NONE',  ( 193.3006371371548369, 56.51400776751751920, 0.000000000000000000 ) ) ;
#6510=ORIENTED_EDGE ( 'NONE', *, *, #681, .T. ) ;
#6512=DIRECTION ( 'NONE',  ( -1.000000000000000000, 0.000000000000000000, 0.000000000000000000 ) ) ;
#6520=VERTEX_POINT ( 'NONE', #6272 ) ;
#6521=FACE_OUTER_BOUND ( 'NONE', #7437, .T. ) ;
#6544=DIRECTION ( 'NONE',  ( -0.000000000000000000, -0.000000000000000000, 1.000000000000000000 ) ) ;
#6547=AXIS2_PLACEMENT_3D ( 'NONE', #8205, #825, #5659 ) ;
#6553=CARTESIAN_POINT ( 'NONE',  ( 190.2479883433758800, 63.36949047362622167, 5.000000000000000000 ) ) ;
#6584=ORIENTED_EDGE ( 'NONE', *, *, #7385, .F. ) ;
#6585=DIRECTION ( 'NONE',  ( 0.8731965799097686221, -0.4873681696970812438, -0.000000000000000000 ) ) ;
#6593=ORIENTED_EDGE ( 'NONE', *, *, #380, .T. ) ;
#6602=FACE_OUTER_BOUND ( 'NONE', #9506, .T. ) ;
#6648=DIRECTION ( 'NONE',  ( -0.000000000000000000, -0.000000000000000000, 1.000000000000000000 ) ) ;
#6663=ORIENTED_EDGE ( 'NONE', *, *, #5376, .F. ) ;
#6670=CYLINDRICAL_SURFACE ( 'NONE', #9553, 10.97218105532926558 ) ;
#6677=DIRECTION ( 'NONE',  ( 1.000000000000000000, 0.000000000000000000, 0.000000000000000000 ) ) ;
#6694=ADVANCED_FACE ( 'NONE', ( #11713 ), #12646, .T. ) ;
#6698=DIRECTION ( 'NONE',  ( 0.8950274278067241740, -0.4460111024107797362, 0.000000000000000000 ) ) ;
#6707=CARTESIAN_POINT ( 'NONE',  ( -144.0627431139473345, 95.36268816863731956, 0.000000000000000000 ) ) ;
#6722=LINE ( 'NONE', #13802, #11076 ) ;
#6751=FACE_OUTER_BOUND ( 'NONE', #15117, .T. ) ;
#6783=FACE_OUTER_BOUND ( 'NONE', #9493, .T. ) ;
#6790=CARTESIAN_POINT ( 'NONE',  ( -85.27455057502459113, 65.19100426474074084, 0.000000000000000000 ) ) ;
#6802=DIRECTION ( 'NONE',  ( 1.000000000000000000, 0.000000000000000000, 0.000000000000000000 ) ) ;
#6814=LINE ( 'NONE', #15157, #7794 ) ;
#6835=ORIENTED_EDGE ( 'NONE', *, *, #895, .T. ) ;
#6842=EDGE_CURVE ( 'NONE', #13988, #7301, #15609, .T. ) ;
#6855=CIRCLE ( 'NONE', #9131, 1.699999999999993072 ) ;
#6856=EDGE_CURVE ( 'NONE', #1071, #4418, #12347, .T. ) ;
#6875=EDGE_LOOP ( 'NONE', ( #8779, #5348, #7994, #8868, #8910, #1593, #2367, #2377, #15320, #13256, #12084, #5427, #7001, #5795 ) ) ;
#6889=DIRECTION ( 'NONE',  ( -0.000000000000000000, -0.000000000000000000, 1.000000000000000000 ) ) ;
#6894=ORIENTED_EDGE ( 'NONE', *, *, #13184, .F. ) ;
#6897=EDGE_CURVE ( 'NONE', #13949, #11700, #12850, .T. ) ;
#6904=AXIS2_PLACEMENT_3D ( 'NONE', #15208, #2114, #15278 ) ;
#6919=CYLINDRICAL_SURFACE ( 'NONE', #5942, 1.700000000000000178 ) ;
#6922=EDGE_LOOP ( 'NONE', ( #12705, #5023, #1877, #2705 ) ) ;
#6946=DIRECTION ( 'NONE',  ( 1.000000000000000000, 0.000000000000000000, 0.000000000000000000 ) ) ;
#6975=DIRECTION ( 'NONE',  ( -0.000000000000000000, -0.000000000000000000, -1.000000000000000000 ) ) ;
#6976=ORIENTED_EDGE ( 'NONE', *, *, #12580, .T. ) ;
#6987=LINE ( 'NONE', #1046, #4670 ) ;
#6989=DIRECTION ( 'NONE',  ( 1.000000000000000000, 0.000000000000000000, 0.000000000000000000 ) ) ;
#6998=VERTEX_POINT ( 'NONE', #8668 ) ;
#7001=ORIENTED_EDGE ( 'NONE', *, *, #895, .F. ) ;
#7023=DIRECTION ( 'NONE',  ( -1.000000000000000000, 0.000000000000000000, 0.000000000000000000 ) ) ;
#7041=SHAPE_REPRESENTATION ( 'Long Manual Lever Operating Handle', ( #12337 ), #6268 ) ;
#7078=VECTOR ( 'NONE', #13830, 1000.000000000000000 ) ;
#7079=ORIENTED_EDGE ( 'NONE', *, *, #4595, .T. ) ;
#7111=DIRECTION ( 'NONE',  ( 1.000000000000000000, 0.000000000000000000, 0.000000000000000000 ) ) ;
#7114=LINE ( 'NONE', #12775, #565 ) ;
#7121=ORIENTED_EDGE ( 'NONE', *, *, #9816, .T. ) ;
#7135=EDGE_LOOP ( 'NONE', ( #3925, #10122, #11133, #7491 ) ) ;
#7140=ORIENTED_EDGE ( 'NONE', *, *, #6842, .F. ) ;
#7148=ORIENTED_EDGE ( 'NONE', *, *, #13825, .F. ) ;
#7157=EDGE_CURVE ( 'NONE', #3263, #1447, #14791, .T. ) ;
#7165=CARTESIAN_POINT ( 'NONE',  ( 15.71029453487719074, 40.04259805664093363, 10.00000000000000178 ) ) ;
#7177=CYLINDRICAL_SURFACE ( 'NONE', #4790, 1.500000000000001332 ) ;
#7193=ADVANCED_FACE ( 'NONE', ( #11262 ), #8027, .F. ) ;
#7195=ORIENTED_EDGE ( 'NONE', *, *, #9811, .T. ) ;
#7201=DIRECTION ( 'NONE',  ( -0.000000000000000000, -0.000000000000000000, -1.000000000000000000 ) ) ;
#7235=CARTESIAN_POINT ( 'NONE',  ( -130.0135953313997561, 106.9229804370480537, 0.000000000000000000 ) ) ;
#7242=DIRECTION ( 'NONE',  ( -0.000000000000000000, -0.000000000000000000, -1.000000000000000000 ) ) ;
#7246=CARTESIAN_POINT ( 'NONE',  ( 200.1062858801516597, 40.86394065090267702, 5.000000000000000000 ) ) ;
#7267=DIRECTION ( 'NONE',  ( 1.000000000000000000, 0.000000000000000000, 0.000000000000000000 ) ) ;
#7272=CARTESIAN_POINT ( 'NONE',  ( 200.1062858801516597, 40.86394065090267702, 0.000000000000000000 ) ) ;
#7299=AXIS2_PLACEMENT_3D ( 'NONE', #13442, #2640, #3589 ) ;
#7301=VERTEX_POINT ( 'NONE', #14160 ) ;
#7307=CARTESIAN_POINT ( 'NONE',  ( 13.07968152355895874, 460.3807876674321165, 0.000000000000000000 ) ) ;
#7312=VECTOR ( 'NONE', #9505, 1000.000000000000000 ) ;
#7313=ORIENTED_EDGE ( 'NONE', *, *, #12226, .F. ) ;
#7353=CARTESIAN_POINT ( 'NONE',  ( 17.41029453487719181, 40.04259805664093363, 0.000000000000000000 ) ) ;
#7358=EDGE_CURVE ( 'NONE', #13697, #14280, #8801, .T. ) ;
#7385=EDGE_CURVE ( 'NONE', #2732, #11374, #4768, .T. ) ;
#7387=ORIENTED_EDGE ( 'NONE', *, *, #7802, .F. ) ;
#7394=EDGE_CURVE ( 'NONE', #8350, #12412, #3019, .T. ) ;
#7411=CARTESIAN_POINT ( 'NONE',  ( 172.5293059057019889, 61.25683321636181233, 0.000000000000000000 ) ) ;
#7420=CARTESIAN_POINT ( 'NONE',  ( 51.07686401294030532, 368.7106150007013525, 5.000000000000000000 ) ) ;
#7437=EDGE_LOOP ( 'NONE', ( #13822, #9100, #4483, #8609 ) ) ;
#7439=CARTESIAN_POINT ( 'NONE',  ( -130.0135953313997561, 106.9229804370480537, 5.000000000000000000 ) ) ;
#7449=PRESENTATION_STYLE_ASSIGNMENT (( #14685 ) ) ;
#7450=ORIENTED_EDGE ( 'NONE', *, *, #1397, .F. ) ;
#7477=EDGE_LOOP ( 'NONE', ( #12176, #4081 ) ) ;
#7491=ORIENTED_EDGE ( 'NONE', *, *, #9969, .T. ) ;
#7511=CARTESIAN_POINT ( 'NONE',  ( 51.07686401294030532, 368.7106150007013525, 5.000000000000000000 ) ) ;
#7514=ORIENTED_EDGE ( 'NONE', *, *, #14792, .T. ) ;
#7539=DIRECTION ( 'NONE',  ( 1.000000000000000000, 0.000000000000000000, 0.000000000000000000 ) ) ;
#7558=AXIS2_PLACEMENT_3D ( 'NONE', #5873, #8257, #6989 ) ;
#7560=DIRECTION ( 'NONE',  ( 1.000000000000000000, 0.000000000000000000, 0.000000000000000000 ) ) ;
#7568=EDGE_LOOP ( 'NONE', ( #32, #10944, #14925, #5467 ) ) ;
#7576=CIRCLE ( 'NONE', #13089, 1.000000000000000888 ) ;
#7602=EDGE_LOOP ( 'NONE', ( #13510, #8501, #2559, #10727 ) ) ;
#7620=DIRECTION ( 'NONE',  ( -0.09810338464376283651, -0.9951762285753403825, 0.000000000000000000 ) ) ;
#7622=DIRECTION ( 'NONE',  ( -0.8731965799097686221, 0.4873681696970811883, 0.000000000000000000 ) ) ;
#7625=ADVANCED_FACE ( 'NONE', ( #12649 ), #3968, .F. ) ;
#7626=VECTOR ( 'NONE', #4734, 1000.000000000000000 ) ;
#7628=CARTESIAN_POINT ( 'NONE',  ( 172.5293059057019889, 61.25683321636181233, 10.00000000000000178 ) ) ;
#7670=VECTOR ( 'NONE', #12207, 1000.000000000000000 ) ;
#7701=ADVANCED_FACE ( 'NONE', ( #5779 ), #14142, .T. ) ;
#7706=AXIS2_PLACEMENT_3D ( 'NONE', #15261, #11419, #6698 ) ;
#7708=ORIENTED_EDGE ( 'NONE', *, *, #4858, .F. ) ;
#7709=DIRECTION ( 'NONE',  ( -0.000000000000000000, -0.000000000000000000, 1.000000000000000000 ) ) ;
#7772=CARTESIAN_POINT ( 'NONE',  ( 215.4200305399390345, 33.33196348269225240, 5.000000000000000000 ) ) ;
#7794=VECTOR ( 'NONE', #13985, 1000.000000000000000 ) ;
#7795=DIRECTION ( 'NONE',  ( 1.000000000000000000, 0.000000000000000000, 0.000000000000000000 ) ) ;
#7802=EDGE_CURVE ( 'NONE', #14996, #5691, #1247, .T. ) ;
#7821=CARTESIAN_POINT ( 'NONE',  ( -155.6477983077465410, 110.1970436846185066, 5.000000000000000000 ) ) ;
#7837=ORIENTED_EDGE ( 'NONE', *, *, #4858, .T. ) ;
#7844=AXIS2_PLACEMENT_3D ( 'NONE', #15133, #14107, #4324 ) ;
#7845=ORIENTED_EDGE ( 'NONE', *, *, #6120, .T. ) ;
#7852=ORIENTED_EDGE ( 'NONE', *, *, #4595, .F. ) ;
#7892=ORIENTED_EDGE ( 'NONE', *, *, #14841, .T. ) ;
#7929=ORIENTED_EDGE ( 'NONE', *, *, #3059, .F. ) ;
#7938=DIRECTION ( 'NONE',  ( -0.000000000000000000, -0.000000000000000000, -1.000000000000000000 ) ) ;
#7943=CIRCLE ( 'NONE', #11965, 1.000000000000000888 ) ;
#7945=DIRECTION ( 'NONE',  ( 0.000000000000000000, 0.000000000000000000, 1.000000000000000000 ) ) ;
#7966=ORIENTED_EDGE ( 'NONE', *, *, #11533, .T. ) ;
#7984=VERTEX_POINT ( 'NONE', #8324 ) ;
#7992=AXIS2_PLACEMENT_3D ( 'NONE', #9695, #1153, #9531 ) ;
#7994=ORIENTED_EDGE ( 'NONE', *, *, #9954, .F. ) ;
#7998=ORIENTED_EDGE ( 'NONE', *, *, #916, .F. ) ;
#8017=CYLINDRICAL_SURFACE ( 'NONE', #6454, 1.700000000000007061 ) ;
#8027=CYLINDRICAL_SURFACE ( 'NONE', #2542, 9.999999999999994671 ) ;
#8038=DIRECTION ( 'NONE',  ( 1.000000000000000000, 0.000000000000000000, 0.000000000000000000 ) ) ;
#8061=VERTEX_POINT ( 'NONE', #6495 ) ;
#8077=CIRCLE ( 'NONE', #6048, 1.700000000000007061 ) ;
#8118=ORIENTED_EDGE ( 'NONE', *, *, #15476, .F. ) ;
#8138=LINE ( 'NONE', #13959, #9670 ) ;
#8141=CIRCLE ( 'NONE', #1303, 59.90987050789675550 ) ;
#8147=DIRECTION ( 'NONE',  ( 0.000000000000000000, 0.000000000000000000, 1.000000000000000000 ) ) ;
#8152=AXIS2_PLACEMENT_3D ( 'NONE', #6042, #3511, #8269 ) ;
#8192=ADVANCED_FACE ( 'NONE', ( #3090 ), #3161, .F. ) ;
#8205=CARTESIAN_POINT ( 'NONE',  ( -130.9946291778373961, 96.97121815129470690, 0.000000000000000000 ) ) ;
#8208=EDGE_CURVE ( 'NONE', #1269, #4524, #6398, .T. ) ;
#8225=DIRECTION ( 'NONE',  ( 0.000000000000000000, 0.000000000000000000, 1.000000000000000000 ) ) ;
#8230=ORIENTED_EDGE ( 'NONE', *, *, #5337, .F. ) ;
#8247=DIRECTION ( 'NONE',  ( -0.000000000000000000, -0.000000000000000000, 1.000000000000000000 ) ) ;
#8254=ORIENTED_EDGE ( 'NONE', *, *, #14587, .F. ) ;
#8257=DIRECTION ( 'NONE',  ( 0.000000000000000000, 0.000000000000000000, 1.000000000000000000 ) ) ;
#8268=EDGE_CURVE ( 'NONE', #1469, #6998, #2752, .T. ) ;
#8269=DIRECTION ( 'NONE',  ( -1.000000000000000000, 0.000000000000000000, 0.000000000000000000 ) ) ;
#8282=DIRECTION ( 'NONE',  ( -0.000000000000000000, -0.000000000000000000, 1.000000000000000000 ) ) ;
#8286=AXIS2_PLACEMENT_3D ( 'NONE', #2033, #3307, #6946 ) ;
#8291=DIRECTION ( 'NONE',  ( 1.000000000000000000, 0.000000000000000000, 0.000000000000000000 ) ) ;
#8296=LINE ( 'NONE', #11834, #11400 ) ;
#8300=FACE_OUTER_BOUND ( 'NONE', #14886, .T. ) ;
#8309=CIRCLE ( 'NONE', #3495, 1.700000000000007061 ) ;
#8313=ORIENTED_EDGE ( 'NONE', *, *, #15238, .F. ) ;
#8317=ORIENTED_EDGE ( 'NONE', *, *, #3303, .F. ) ;
#8324=CARTESIAN_POINT ( 'NONE',  ( -164.5262273476079713, 106.7842295329138835, 0.000000000000000000 ) ) ;
#8329=DIRECTION ( 'NONE',  ( -0.000000000000000000, -0.000000000000000000, 1.000000000000000000 ) ) ;
#8337=COLOUR_RGB ( '', 0.08235294, 0.09019608, 0.10196078) ;
#8341=FACE_BOUND ( 'NONE', #7477, .T. ) ;
#8350=VERTEX_POINT ( 'NONE', #6308 ) ;
#8359=VECTOR ( 'NONE', #12856, 1000.000000000000000 ) ;
#8360=FACE_OUTER_BOUND ( 'NONE', #3957, .T. ) ;
#8403=DIRECTION ( 'NONE',  ( 0.000000000000000000, 0.000000000000000000, 1.000000000000000000 ) ) ;
#8430=CARTESIAN_POINT ( 'NONE',  ( -144.0627431139473345, 95.36268816863731956, 5.000000000000000000 ) ) ;
#8452=DIRECTION ( 'NONE',  ( 1.000000000000000000, 0.000000000000000000, 0.000000000000000000 ) ) ;
#8456=CARTESIAN_POINT ( 'NONE',  ( 17.41029453487719181, 40.04259805664093363, 0.000000000000000000 ) ) ;
#8460=CARTESIAN_POINT ( 'NONE',  ( -83.77455057502459113, 65.19100426474074084, -20.00000000000000000 ) ) ;
#8485=AXIS2_PLACEMENT_3D ( 'NONE', #11883, #15489, #13199 ) ;
#8490=ORIENTED_EDGE ( 'NONE', *, *, #2938, .T. ) ;
#8494=FACE_BOUND ( 'NONE', #2180, .T. ) ;
#8498=EDGE_CURVE ( 'NONE', #7984, #6369, #9299, .T. ) ;
#8501=ORIENTED_EDGE ( 'NONE', *, *, #15293, .F. ) ;
#8525=VECTOR ( 'NONE', #13615, 1000.000000000000000 ) ;
#8567=ADVANCED_FACE ( 'NONE', ( #12755 ), #11586, .F. ) ;
#8585=VERTEX_POINT ( 'NONE', #2419 ) ;
#8591=VECTOR ( 'NONE', #9767, 1000.000000000000000 ) ;
#8609=ORIENTED_EDGE ( 'NONE', *, *, #4340, .F. ) ;
#8629=CYLINDRICAL_SURFACE ( 'NONE', #14964, 1.700000000000007061 ) ;
#8634=EDGE_CURVE ( 'NONE', #3314, #4605, #14408, .T. ) ;
#8656=ADVANCED_FACE ( 'NONE', ( #8360 ), #106, .F. ) ;
#8663=ORIENTED_EDGE ( 'NONE', *, *, #4851, .T. ) ;
#8668=CARTESIAN_POINT ( 'NONE',  ( -86.77455057502459113, 65.19100426474074084, 5.000000000000000000 ) ) ;
#8676=DIRECTION ( 'NONE',  ( -1.000000000000000000, 0.000000000000000000, 0.000000000000000000 ) ) ;
#8677=ORIENTED_EDGE ( 'NONE', *, *, #1163, .F. ) ;
#8688=CIRCLE ( 'NONE', #12946, 1.700000000000000178 ) ;
#8695=ORIENTED_EDGE ( 'NONE', *, *, #13511, .F. ) ;
#8700=EDGE_LOOP ( 'NONE', ( #7387, #7514, #13742, #4479 ) ) ;
#8723=AXIS2_PLACEMENT_3D ( 'NONE', #9748, #11010, #7622 ) ;
#8779=ORIENTED_EDGE ( 'NONE', *, *, #10114, .F. ) ;
#8801=CIRCLE ( 'NONE', #7299, 17.06579782980005433 ) ;
#8816=ADVANCED_FACE ( 'NONE', ( #11681, #11521, #11756, #15049, #9081, #679, #9313, #844, #5523, #3382 ), #4477, .T. ) ;
#8821=AXIS2_PLACEMENT_3D ( 'NONE', #5709, #7938, #3339 ) ;
#8854=DIRECTION ( 'NONE',  ( 0.000000000000000000, 0.000000000000000000, 1.000000000000000000 ) ) ;
#8868=ORIENTED_EDGE ( 'NONE', *, *, #12783, .F. ) ;
#8879=CARTESIAN_POINT ( 'NONE',  ( 195.1062858801516597, 40.86394065090267702, -20.00000000000000000 ) ) ;
#8885=APPLICATION_CONTEXT ( 'automotive_design' ) ;
#8891=DIRECTION ( 'NONE',  ( -0.000000000000000000, -0.000000000000000000, -1.000000000000000000 ) ) ;
#8910=ORIENTED_EDGE ( 'NONE', *, *, #11356, .F. ) ;
#8915=DIRECTION ( 'NONE',  ( -0.000000000000000000, -0.000000000000000000, 1.000000000000000000 ) ) ;
#8939=EDGE_CURVE ( 'NONE', #14692, #1447, #10096, .T. ) ;
#8968=DIRECTION ( 'NONE',  ( 1.000000000000000000, 0.000000000000000000, 0.000000000000000000 ) ) ;
#8979=DIRECTION ( 'NONE',  ( 1.000000000000000000, 0.000000000000000000, 0.000000000000000000 ) ) ;
#9000=AXIS2_PLACEMENT_3D ( 'NONE', #15588, #11982, #14329 ) ;
#9004=CARTESIAN_POINT ( 'NONE',  ( -173.4445345933175986, 43.15250799526725700, 0.000000000000000000 ) ) ;
#9027=DIRECTION ( 'NONE',  ( -0.000000000000000000, -0.000000000000000000, -1.000000000000000000 ) ) ;
#9062=CYLINDRICAL_SURFACE ( 'NONE', #4523, 1.000000000000000888 ) ;
#9081=FACE_BOUND ( 'NONE', #1388, .T. ) ;
#9096=ORIENTED_EDGE ( 'NONE', *, *, #15476, .T. ) ;
#9100=ORIENTED_EDGE ( 'NONE', *, *, #15100, .T. ) ;
#9104=DIRECTION ( 'NONE',  ( -0.000000000000000000, -0.000000000000000000, -1.000000000000000000 ) ) ;
#9120=DIRECTION ( 'NONE',  ( 0.000000000000000000, 0.000000000000000000, 1.000000000000000000 ) ) ;
#9122=ORIENTED_EDGE ( 'NONE', *, *, #2967, .F. ) ;
#9131=AXIS2_PLACEMENT_3D ( 'NONE', #4589, #8403, #13254 ) ;
#9148=ORIENTED_EDGE ( 'NONE', *, *, #10921, .T. ) ;
#9153=DIRECTION ( 'NONE',  ( -0.000000000000000000, -0.000000000000000000, 1.000000000000000000 ) ) ;
#9159=EDGE_CURVE ( 'NONE', #8585, #555, #11365, .T. ) ;
#9169=VECTOR ( 'NONE', #8915, 1000.000000000000000 ) ;
#9176=DIRECTION ( 'NONE',  ( 1.000000000000000000, 0.000000000000000000, 0.000000000000000000 ) ) ;
#9182=CARTESIAN_POINT ( 'NONE',  ( -173.4445345933175986, 43.15250799526725700, 5.000000000000000000 ) ) ;
#9294=EDGE_LOOP ( 'NONE', ( #9122, #14511 ) ) ;
#9299=LINE ( 'NONE', #6707, #10781 ) ;
#9308=VECTOR ( 'NONE', #6648, 1000.000000000000000 ) ;
#9309=DIRECTION ( 'NONE',  ( -0.000000000000000000, -0.000000000000000000, -1.000000000000000000 ) ) ;
#9313=FACE_BOUND ( 'NONE', #13169, .T. ) ;
#9364=EDGE_CURVE ( 'NONE', #555, #8585, #4805, .T. ) ;
#9377=ORIENTED_EDGE ( 'NONE', *, *, #15360, .F. ) ;
#9381=CARTESIAN_POINT ( 'NONE',  ( -155.6477983077465410, 110.1970436846185066, 0.000000000000000000 ) ) ;
#9385=CARTESIAN_POINT ( 'NONE',  ( 200.1062858801516597, 40.86394065090267702, -20.00000000000000000 ) ) ;
#9407=CARTESIAN_POINT ( 'NONE',  ( 172.5293059057019889, 61.25683321636181233, 5.000000000000000000 ) ) ;
#9411=CARTESIAN_POINT ( 'NONE',  ( 169.5018791832601721, 101.0521538385604003, 5.000000000000000000 ) ) ;
#9431=ADVANCED_BREP_SHAPE_REPRESENTATION ( '', ( #11106, #12337 ), #6268 ) ;
#9443=AXIS2_PLACEMENT_3D ( 'NONE', #11299, #4475, #7023 ) ;
#9457=DIRECTION ( 'NONE',  ( 0.000000000000000000, 0.000000000000000000, 1.000000000000000000 ) ) ;
#9478=ORIENTED_EDGE ( 'NONE', *, *, #10921, .F. ) ;
#9493=EDGE_LOOP ( 'NONE', ( #7450, #9377, #3603, #9608 ) ) ;
#9500=DIRECTION ( 'NONE',  ( 1.000000000000000000, 0.000000000000000000, 0.000000000000000000 ) ) ;
#9505=DIRECTION ( 'NONE',  ( -0.000000000000000000, -0.000000000000000000, 1.000000000000000000 ) ) ;
#9506=EDGE_LOOP ( 'NONE', ( #1977, #10571, #10210, #667 ) ) ;
#9510=FACE_BOUND ( 'NONE', #1644, .T. ) ;
#9523=DIRECTION ( 'NONE',  ( -0.000000000000000000, -0.000000000000000000, 1.000000000000000000 ) ) ;
#9531=DIRECTION ( 'NONE',  ( 1.000000000000000000, 0.000000000000000000, 0.000000000000000000 ) ) ;
#9534=DIRECTION ( 'NONE',  ( 1.000000000000000000, 0.000000000000000000, 0.000000000000000000 ) ) ;
#9553=AXIS2_PLACEMENT_3D ( 'NONE', #9411, #14209, #10443 ) ;
#9576=LINE ( 'NONE', #9658, #13798 ) ;
#9578=CARTESIAN_POINT ( 'NONE',  ( 200.1062858801516597, 40.86394065090267702, -20.00000000000000000 ) ) ;
#9608=ORIENTED_EDGE ( 'NONE', *, *, #15132, .T. ) ;
#9632=CARTESIAN_POINT ( 'NONE',  ( 193.3006371371548369, 56.51400776751751920, 5.000000000000000000 ) ) ;
#9634=DIRECTION ( 'NONE',  ( 0.000000000000000000, 0.000000000000000000, 1.000000000000000000 ) ) ;
#9658=CARTESIAN_POINT ( 'NONE',  ( -157.8787660911425803, 118.6941998492684149, 5.000000000000000000 ) ) ;
#9663=LINE ( 'NONE', #4998, #4515 ) ;
#9665=ORIENTED_EDGE ( 'NONE', *, *, #12580, .F. ) ;
#9670=VECTOR ( 'NONE', #3304, 1000.000000000000000 ) ;
#9687=AXIS2_PLACEMENT_3D ( 'NONE', #9694, #11028, #1152 ) ;
#9694=CARTESIAN_POINT ( 'NONE',  ( -85.27455057502459113, 65.19100426474074084, 5.000000000000000000 ) ) ;
#9695=CARTESIAN_POINT ( 'NONE',  ( 70.26535645333922275, 38.79159067395544014, 0.000000000000000000 ) ) ;
#9709=DIRECTION ( 'NONE',  ( 0.000000000000000000, 0.000000000000000000, 1.000000000000000000 ) ) ;
#9728=DIRECTION ( 'NONE',  ( -0.000000000000000000, -0.000000000000000000, -1.000000000000000000 ) ) ;
#9735=SURFACE_STYLE_FILL_AREA ( #3810 ) ;
#9737=ORIENTED_EDGE ( 'NONE', *, *, #10291, .F. ) ;
#9738=CIRCLE ( 'NONE', #8485, 5.000000000000004441 ) ;
#9748=CARTESIAN_POINT ( 'NONE',  ( -144.0627431139473345, 95.36268816863731956, 5.000000000000000000 ) ) ;
#9751=CIRCLE ( 'NONE', #2944, 59.90987050789675550 ) ;
#9757=LINE ( 'NONE', #7165, #10893 ) ;
#9766=DIRECTION ( 'NONE',  ( -1.000000000000000000, 0.000000000000000000, 0.000000000000000000 ) ) ;
#9767=DIRECTION ( 'NONE',  ( -0.000000000000000000, -0.000000000000000000, -1.000000000000000000 ) ) ;
#9772=CARTESIAN_POINT ( 'NONE',  ( 68.56535645333921991, 38.79159067395544014, 10.00000000000000178 ) ) ;
#9773=CARTESIAN_POINT ( 'NONE',  ( -156.6477983077465410, 110.1970436846185066, 0.000000000000000000 ) ) ;
#9790=AXIS2_PLACEMENT_3D ( 'NONE', #8456, #9709, #7267 ) ;
#9810=EDGE_CURVE ( 'NONE', #12123, #13122, #13180, .T. ) ;
#9811=EDGE_CURVE ( 'NONE', #6520, #8350, #3409, .T. ) ;
#9816=EDGE_CURVE ( 'NONE', #12412, #8061, #2034, .T. ) ;
#9822=ORIENTED_EDGE ( 'NONE', *, *, #5987, .T. ) ;
#9826=VERTEX_POINT ( 'NONE', #14288 ) ;
#9829=AXIS2_PLACEMENT_3D ( 'NONE', #7307, #4764, #2474 ) ;
#9832=AXIS2_PLACEMENT_3D ( 'NONE', #13003, #14114, #14188 ) ;
#9851=ORIENTED_EDGE ( 'NONE', *, *, #839, .T. ) ;
#9857=VECTOR ( 'NONE', #14253, 1000.000000000000000 ) ;
#9893=ORIENTED_EDGE ( 'NONE', *, *, #4851, .F. ) ;
#9914=EDGE_LOOP ( 'NONE', ( #4936, #4248, #10663, #2946 ) ) ;
#9915=DIRECTION ( 'NONE',  ( -0.000000000000000000, 0.000000000000000000, 1.000000000000000000 ) ) ;
#9925=EDGE_CURVE ( 'NONE', #4605, #10761, #6855, .T. ) ;
#9953=LINE ( 'NONE', #5205, #14946 ) ;
#9954=EDGE_CURVE ( 'NONE', #10673, #3263, #3827, .T. ) ;
#9969=EDGE_CURVE ( 'NONE', #1126, #3245, #2615, .T. ) ;
#10003=ORIENTED_EDGE ( 'NONE', *, *, #392, .T. ) ;
#10007=DIRECTION ( 'NONE',  ( 0.000000000000000000, 0.000000000000000000, 1.000000000000000000 ) ) ;
#10016=CARTESIAN_POINT ( 'NONE',  ( -34.79899788034579444, 48.72489408690345414, 0.000000000000000000 ) ) ;
#10050=ORIENTED_EDGE ( 'NONE', *, *, #11037, .T. ) ;
#10082=ORIENTED_EDGE ( 'NONE', *, *, #13862, .F. ) ;
#10096=CIRCLE ( 'NONE', #3282, 380.9270036976043343 ) ;
#10108=CARTESIAN_POINT ( 'NONE',  ( -157.8787660911425803, 118.6941998492684149, 5.000000000000000000 ) ) ;
#10109=ORIENTED_EDGE ( 'NONE', *, *, #13862, .T. ) ;
#10114=EDGE_CURVE ( 'NONE', #3245, #12123, #13728, .T. ) ;
#10122=ORIENTED_EDGE ( 'NONE', *, *, #9810, .T. ) ;
#10138=CARTESIAN_POINT ( 'NONE',  ( 166.3583383998781358, 57.46267437295986014, 5.000000000000000000 ) ) ;
#10145=EDGE_LOOP ( 'NONE', ( #2129, #4137, #3719, #12949 ) ) ;
#10147=DIRECTION ( 'NONE',  ( -0.000000000000000000, -0.000000000000000000, 1.000000000000000000 ) ) ;
#10159=CARTESIAN_POINT ( 'NONE',  ( 165.1224552381025887, 111.1124422548786299, 0.000000000000000000 ) ) ;
#10210=ORIENTED_EDGE ( 'NONE', *, *, #4340, .T. ) ;
#10216=DIRECTION ( 'NONE',  ( -0.000000000000000000, -0.000000000000000000, -1.000000000000000000 ) ) ;
#10230=VECTOR ( 'NONE', #6585, 1000.000000000000000 ) ;
#10244=DIRECTION ( 'NONE',  ( 1.000000000000000000, 0.000000000000000000, 0.000000000000000000 ) ) ;
#10255=CARTESIAN_POINT ( 'NONE',  ( -85.27455057502459113, 65.19100426474074084, -20.00000000000000000 ) ) ;
#10291=EDGE_CURVE ( 'NONE', #6229, #1785, #13645, .T. ) ;
#10306=ORIENTED_EDGE ( 'NONE', *, *, #6120, .F. ) ;
#10323=AXIS2_PLACEMENT_3D ( 'NONE', #14842, #4037, #13741 ) ;
#10338=AXIS2_PLACEMENT_3D ( 'NONE', #14325, #9457, #14254 ) ;
#10363=AXIS2_PLACEMENT_3D ( 'NONE', #5736, #10479, #10244 ) ;
#10374=ORIENTED_EDGE ( 'NONE', *, *, #7358, .T. ) ;
#10401=ORIENTED_EDGE ( 'NONE', *, *, #2770, .T. ) ;
#10413=FACE_OUTER_BOUND ( 'NONE', #15116, .T. ) ;
#10443=DIRECTION ( 'NONE',  ( -1.000000000000000000, 0.000000000000000000, 0.000000000000000000 ) ) ;
#10453=DIRECTION ( 'NONE',  ( 0.000000000000000000, 0.000000000000000000, 1.000000000000000000 ) ) ;
#10456=PLANE ( 'NONE',  #15492 ) ;
#10479=DIRECTION ( 'NONE',  ( 0.000000000000000000, 0.000000000000000000, 1.000000000000000000 ) ) ;
#10499=LINE ( 'NONE', #15137, #9308 ) ;
#10551=EDGE_LOOP ( 'NONE', ( #7852, #6593, #11310, #1174 ) ) ;
#10571=ORIENTED_EDGE ( 'NONE', *, *, #11533, .F. ) ;
#10574=PRODUCT_DEFINITION ( 'UNKNOWN', '', #6024, #12612 ) ;
#10580=DIRECTION ( 'NONE',  ( -0.000000000000000000, -0.000000000000000000, 1.000000000000000000 ) ) ;
#10589=EDGE_LOOP ( 'NONE', ( #12120, #12328, #6510, #14510 ) ) ;
#10598=ORIENTED_EDGE ( 'NONE', *, *, #518, .T. ) ;
#10601=ORIENTED_EDGE ( 'NONE', *, *, #7394, .T. ) ;
#10620=CARTESIAN_POINT ( 'NONE',  ( -33.09899788034579871, 48.72489408690345414, 0.000000000000000000 ) ) ;
#10627=ORIENTED_EDGE ( 'NONE', *, *, #12307, .T. ) ;
#10656=DIRECTION ( 'NONE',  ( -0.000000000000000000, -0.000000000000000000, 1.000000000000000000 ) ) ;
#10657=CARTESIAN_POINT ( 'NONE',  ( 122.5806775638430253, 45.00321902537314145, 5.000000000000000000 ) ) ;
#10663=ORIENTED_EDGE ( 'NONE', *, *, #14711, .F. ) ;
#10673=VERTEX_POINT ( 'NONE', #10159 ) ;
#10681=AXIS2_PLACEMENT_3D ( 'NONE', #10255, #12611, #603 ) ;
#10696=ORIENTED_EDGE ( 'NONE', *, *, #401, .F. ) ;
#10700=DIRECTION ( 'NONE',  ( 0.000000000000000000, 0.000000000000000000, 1.000000000000000000 ) ) ;
#10725=CARTESIAN_POINT ( 'NONE',  ( 71.96535645333923981, 38.79159067395544014, 5.000000000000000000 ) ) ;
#10727=ORIENTED_EDGE ( 'NONE', *, *, #9925, .T. ) ;
#10728=SHAPE_REPRESENTATION_RELATIONSHIP ( 'NONE' , 'NONE' ,  #7041, #9431 ) ;
#10731=CARTESIAN_POINT ( 'NONE',  ( 124.2806775638430281, 45.00321902537314145, 0.000000000000000000 ) ) ;
#10741=EDGE_CURVE ( 'NONE', #1584, #13113, #14165, .T. ) ;
#10754=CIRCLE ( 'NONE', #14274, 1.000000000000000888 ) ;
#10761=VERTEX_POINT ( 'NONE', #3435 ) ;
#10781=VECTOR ( 'NONE', #5510, 1000.000000000000000 ) ;
#10802=DIRECTION ( 'NONE',  ( -0.000000000000000000, -0.000000000000000000, 1.000000000000000000 ) ) ;
#10803=CARTESIAN_POINT ( 'NONE',  ( 17.41029453487719181, 40.04259805664093363, 10.00000000000000178 ) ) ;
#10811=ORIENTED_EDGE ( 'NONE', *, *, #2770, .F. ) ;
#10825=CIRCLE ( 'NONE', #11571, 10.97218105532926558 ) ;
#10878=AXIS2_PLACEMENT_3D ( 'NONE', #11455, #539, #4175 ) ;
#10888=EDGE_CURVE ( 'NONE', #2654, #12864, #7576, .T. ) ;
#10893=VECTOR ( 'NONE', #14546, 1000.000000000000000 ) ;
#10921=EDGE_CURVE ( 'NONE', #4524, #1269, #1756, .T. ) ;
#10925=CARTESIAN_POINT ( 'NONE',  ( 70.26535645333922275, 38.79159067395544014, 10.00000000000000178 ) ) ;
#10944=ORIENTED_EDGE ( 'NONE', *, *, #9810, .F. ) ;
#10963=CYLINDRICAL_SURFACE ( 'NONE', #4633, 5.000000000000004441 ) ;
#10972=DIRECTION ( 'NONE',  ( 1.000000000000000000, 0.000000000000000000, 0.000000000000000000 ) ) ;
#10992=ORIENTED_EDGE ( 'NONE', *, *, #4277, .T. ) ;
#11010=DIRECTION ( 'NONE',  ( 0.4873681696970812438, 0.8731965799097687331, -0.000000000000000000 ) ) ;
#11014=ORIENTED_EDGE ( 'NONE', *, *, #14625, .T. ) ;
#11017=DIRECTION ( 'NONE',  ( 1.000000000000000000, 0.000000000000000000, 0.000000000000000000 ) ) ;
#11028=DIRECTION ( 'NONE',  ( -0.000000000000000000, 0.000000000000000000, 1.000000000000000000 ) ) ;
#11037=EDGE_CURVE ( 'NONE', #1785, #6229, #8077, .T. ) ;
#11076=VECTOR ( 'NONE', #3152, 1000.000000000000000 ) ;
#11106=MANIFOLD_SOLID_BREP ( 'Cut-Extrude4', #14647 ) ;
#11108=ORIENTED_EDGE ( 'NONE', *, *, #14841, .F. ) ;
#11109=DIRECTION ( 'NONE',  ( 0.000000000000000000, 0.000000000000000000, 1.000000000000000000 ) ) ;
#11123=ORIENTED_EDGE ( 'NONE', *, *, #2169, .T. ) ;
#11133=ORIENTED_EDGE ( 'NONE', *, *, #12307, .F. ) ;
#11136=ADVANCED_FACE ( 'NONE', ( #13346 ), #8629, .F. ) ;
#11200=CARTESIAN_POINT ( 'NONE',  ( -86.77455057502459113, 65.19100426474074084, -20.00000000000000000 ) ) ;
#11248=CARTESIAN_POINT ( 'NONE',  ( 205.1062858801516597, 40.86394065090267702, -20.00000000000000000 ) ) ;
#11261=DIRECTION ( 'NONE',  ( 1.000000000000000000, 0.000000000000000000, 0.000000000000000000 ) ) ;
#11262=FACE_OUTER_BOUND ( 'NONE', #7568, .T. ) ;
#11264=ORIENTED_EDGE ( 'NONE', *, *, #6842, .T. ) ;
#11299=CARTESIAN_POINT ( 'NONE',  ( 166.3583383998781358, 57.46267437295986014, 0.000000000000000000 ) ) ;
#11310=ORIENTED_EDGE ( 'NONE', *, *, #12226, .T. ) ;
#11320=CARTESIAN_POINT ( 'NONE',  ( -156.6477983077465410, 110.1970436846185066, 5.000000000000000000 ) ) ;
#11330=AXIS2_PLACEMENT_3D ( 'NONE', #6191, #3578, #14614 ) ;
#11343=DIRECTION ( 'NONE',  ( 1.000000000000000000, 0.000000000000000000, 0.000000000000000000 ) ) ;
#11356=EDGE_CURVE ( 'NONE', #14280, #15168, #2887, .T. ) ;
#11359=DIRECTION ( 'NONE',  ( -1.000000000000000000, 0.000000000000000000, 0.000000000000000000 ) ) ;
#11365=CIRCLE ( 'NONE', #2794, 1.700000000000007061 ) ;
#11374=VERTEX_POINT ( 'NONE', #3146 ) ;
#11385=CYLINDRICAL_SURFACE ( 'NONE', #2415, 59.90987050789675550 ) ;
#11387=DIRECTION ( 'NONE',  ( 0.000000000000000000, 0.000000000000000000, 1.000000000000000000 ) ) ;
#11395=CARTESIAN_POINT ( 'NONE',  ( -135.3034657297974093, 107.4444500778096483, 5.000000000000000000 ) ) ;
#11400=VECTOR ( 'NONE', #14186, 1000.000000000000227 ) ;
#11417=CARTESIAN_POINT ( 'NONE',  ( 120.8806775638430224, 45.00321902537314145, 10.00000000000000178 ) ) ;
#11419=DIRECTION ( 'NONE',  ( -0.4460111024107797362, -0.8950274278067241740, 0.000000000000000000 ) ) ;
#11422=CARTESIAN_POINT ( 'NONE',  ( 120.8806775638430224, 45.00321902537314145, 0.000000000000000000 ) ) ;
#11431=DIRECTION ( 'NONE',  ( -0.000000000000000000, -0.000000000000000000, -1.000000000000000000 ) ) ;
#11455=CARTESIAN_POINT ( 'NONE',  ( 200.1062858801516597, 40.86394065090267702, 0.000000000000000000 ) ) ;
#11460=SHAPE_DEFINITION_REPRESENTATION ( #11552, #7041 ) ;
#11468=EDGE_CURVE ( 'NONE', #5691, #14996, #7943, .T. ) ;
#11475=ORIENTED_EDGE ( 'NONE', *, *, #362, .F. ) ;
#11489=ORIENTED_EDGE ( 'NONE', *, *, #1625, .T. ) ;
#11500=LINE ( 'NONE', #11417, #8525 ) ;
#11501=ORIENTED_EDGE ( 'NONE', *, *, #8939, .T. ) ;
#11510=VERTEX_POINT ( 'NONE', #13535 ) ;
#11521=FACE_BOUND ( 'NONE', #13019, .T. ) ;
#11533=EDGE_CURVE ( 'NONE', #4096, #5874, #13472, .T. ) ;
#11552=PRODUCT_DEFINITION_SHAPE ( 'NONE', 'NONE',  #10574 ) ;
#11571=AXIS2_PLACEMENT_3D ( 'NONE', #12827, #902, #3289 ) ;
#11577=AXIS2_PLACEMENT_3D ( 'NONE', #7511, #8854, #6410 ) ;
#11586=CYLINDRICAL_SURFACE ( 'NONE', #5297, 1.700000000000007061 ) ;
#11605=FACE_OUTER_BOUND ( 'NONE', #7602, .T. ) ;
#11626=EDGE_LOOP ( 'NONE', ( #14392, #8254 ) ) ;
#11631=ADVANCED_FACE ( 'NONE', ( #3851 ), #13466, .F. ) ;
#11677=DIRECTION ( 'NONE',  ( -0.000000000000000000, -0.000000000000000000, -1.000000000000000000 ) ) ;
#11681=FACE_BOUND ( 'NONE', #9294, .T. ) ;
#11700=VERTEX_POINT ( 'NONE', #5656 ) ;
#11706=ORIENTED_EDGE ( 'NONE', *, *, #14989, .T. ) ;
#11713=FACE_OUTER_BOUND ( 'NONE', #13886, .T. ) ;
#11727=CARTESIAN_POINT ( 'NONE',  ( 17.41029453487719181, 40.04259805664093363, 10.00000000000000178 ) ) ;
#11756=FACE_BOUND ( 'NONE', #2790, .T. ) ;
#11782=EDGE_LOOP ( 'NONE', ( #15577, #9478, #7837, #2052 ) ) ;
#11796=UNCERTAINTY_MEASURE_WITH_UNIT (LENGTH_MEASURE( 1.000000000000000082E-05 ), #4919, 'distance_accuracy_value', 'NONE');
#11798=CIRCLE ( 'NONE', #8286, 1.700000000000007061 ) ;
#11804=ORIENTED_EDGE ( 'NONE', *, *, #4277, .F. ) ;
#11831=CIRCLE ( 'NONE', #2505, 1.000000000000000888 ) ;
#11834=CARTESIAN_POINT ( 'NONE',  ( -157.8787660911425803, 118.6941998492684149, 0.000000000000000000 ) ) ;
#11837=CYLINDRICAL_SURFACE ( 'NONE', #678, 1.700000000000007061 ) ;
#11851=AXIS2_PLACEMENT_3D ( 'NONE', #876, #7201, #11999 ) ;
#11863=CYLINDRICAL_SURFACE ( 'NONE', #12847, 1.000000000000000888 ) ;
#11877=DIRECTION ( 'NONE',  ( 1.000000000000000000, 0.000000000000000000, 0.000000000000000000 ) ) ;
#11883=CARTESIAN_POINT ( 'NONE',  ( 200.1062858801516597, 40.86394065090267702, 0.000000000000000000 ) ) ;
#11906=AXIS2_PLACEMENT_3D ( 'NONE', #6790, #12690, #680 ) ;
#11913=( NAMED_UNIT ( * ) SI_UNIT ( $, .STERADIAN. ) SOLID_ANGLE_UNIT ( ) );
#11915=DIRECTION ( 'NONE',  ( -0.000000000000000000, -0.000000000000000000, 1.000000000000000000 ) ) ;
#11965=AXIS2_PLACEMENT_3D ( 'NONE', #9773, #14565, #3768 ) ;
#11982=DIRECTION ( 'NONE',  ( 0.000000000000000000, 0.000000000000000000, 1.000000000000000000 ) ) ;
#11983=EDGE_CURVE ( 'NONE', #13122, #14293, #4151, .T. ) ;
#11998=DIRECTION ( 'NONE',  ( -0.000000000000000000, -0.000000000000000000, -1.000000000000000000 ) ) ;
#11999=DIRECTION ( 'NONE',  ( -1.000000000000000000, 0.000000000000000000, 0.000000000000000000 ) ) ;
#12020=CARTESIAN_POINT ( 'NONE',  ( 17.41029453487719181, 40.04259805664093363, 5.000000000000000000 ) ) ;
#12030=CARTESIAN_POINT ( 'NONE',  ( -144.0627431139473345, 95.36268816863731956, 0.000000000000000000 ) ) ;
#12032=ADVANCED_FACE ( 'NONE', ( #6602 ), #8017, .F. ) ;
#12033=DIRECTION ( 'NONE',  ( 0.000000000000000000, 0.000000000000000000, 1.000000000000000000 ) ) ;
#12047=CARTESIAN_POINT ( 'NONE',  ( 191.8042410000843745, 59.95507574834591225, 5.000000000000000000 ) ) ;
#12049=VECTOR ( 'NONE', #11431, 1000.000000000000000 ) ;
#12075=ORIENTED_EDGE ( 'NONE', *, *, #8939, .F. ) ;
#12084=ORIENTED_EDGE ( 'NONE', *, *, #8498, .F. ) ;
#12094=ORIENTED_EDGE ( 'NONE', *, *, #15080, .F. ) ;
#12104=PLANE ( 'NONE',  #9829 ) ;
#12120=ORIENTED_EDGE ( 'NONE', *, *, #14792, .F. ) ;
#12123=VERTEX_POINT ( 'NONE', #1765 ) ;
#12125=AXIS2_PLACEMENT_3D ( 'NONE', #10016, #14797, #8452 ) ;
#12138=VECTOR ( 'NONE', #7242, 1000.000000000000000 ) ;
#12139=FACE_OUTER_BOUND ( 'NONE', #15187, .T. ) ;
#12150=CIRCLE ( 'NONE', #13406, 1.000000000000000888 ) ;
#12152=ADVANCED_FACE ( 'NONE', ( #6751 ), #10456, .F. ) ;
#12175=ORIENTED_EDGE ( 'NONE', *, *, #15293, .T. ) ;
#12176=ORIENTED_EDGE ( 'NONE', *, *, #822, .T. ) ;
#12207=DIRECTION ( 'NONE',  ( -0.000000000000000000, -0.000000000000000000, 1.000000000000000000 ) ) ;
#12226=EDGE_CURVE ( 'NONE', #13651, #4381, #3160, .T. ) ;
#12254=EDGE_LOOP ( 'NONE', ( #11501, #8490, #10627, #13525, #10109, #9096, #215, #79, #10992, #13868, #4014, #7892, #4650, #11014 ) ) ;
#12275=ADVANCED_FACE ( 'NONE', ( #13188 ), #4755, .F. ) ;
#12307=EDGE_CURVE ( 'NONE', #1126, #13122, #6987, .T. ) ;
#12321=FILL_AREA_STYLE_COLOUR ( '', #8337 ) ;
#12328=ORIENTED_EDGE ( 'NONE', *, *, #11468, .F. ) ;
#12337=AXIS2_PLACEMENT_3D ( 'NONE', #4568, #8147, #5681 ) ;
#12347=CIRCLE ( 'NONE', #2009, 1.700000000000000178 ) ;
#12356=DIRECTION ( 'NONE',  ( 1.000000000000000000, 0.000000000000000000, 0.000000000000000000 ) ) ;
#12412=VERTEX_POINT ( 'NONE', #14613 ) ;
#12423=CARTESIAN_POINT ( 'NONE',  ( -157.6477983077465694, 110.1970436846185066, 0.000000000000000000 ) ) ;
#12437=CARTESIAN_POINT ( 'NONE',  ( 172.5293059057019889, 61.25683321636181233, 0.000000000000000000 ) ) ;
#12496=DIRECTION ( 'NONE',  ( 1.000000000000000000, 2.775557561562892929E-15, 0.000000000000000000 ) ) ;
#12524=CARTESIAN_POINT ( 'NONE',  ( -157.6477983077465694, 110.1970436846185066, 5.000000000000000000 ) ) ;
#12529=ADVANCED_FACE ( 'NONE', ( #1895 ), #11385, .F. ) ;
#12561=LINE ( 'NONE', #8879, #7078 ) ;
#12580=EDGE_CURVE ( 'NONE', #10761, #4605, #3415, .T. ) ;
#12581=CARTESIAN_POINT ( 'NONE',  ( -127.3091761562077409, 106.2673160437096413, 5.000000000000000000 ) ) ;
#12611=DIRECTION ( 'NONE',  ( -0.000000000000000000, -0.000000000000000000, 1.000000000000000000 ) ) ;
#12612=PRODUCT_DEFINITION_CONTEXT ( 'detailed design', #8885, 'design' ) ;
#12617=DIRECTION ( 'NONE',  ( -0.000000000000000000, -0.000000000000000000, -1.000000000000000000 ) ) ;
#12630=DIRECTION ( 'NONE',  ( -0.000000000000000000, -0.000000000000000000, 1.000000000000000000 ) ) ;
#12631=VERTEX_POINT ( 'NONE', #4114 ) ;
#12646=CYLINDRICAL_SURFACE ( 'NONE', #11851, 17.06579782980005433 ) ;
#12649=FACE_OUTER_BOUND ( 'NONE', #13271, .T. ) ;
#12661=EDGE_CURVE ( 'NONE', #4947, #3997, #4261, .T. ) ;
#12676=ORIENTED_EDGE ( 'NONE', *, *, #6897, .T. ) ;
#12678=LINE ( 'NONE', #5351, #2733 ) ;
#12690=DIRECTION ( 'NONE',  ( 0.000000000000000000, 0.000000000000000000, 1.000000000000000000 ) ) ;
#12705=ORIENTED_EDGE ( 'NONE', *, *, #13495, .F. ) ;
#12737=FACE_BOUND ( 'NONE', #13423, .T. ) ;
#12740=DIRECTION ( 'NONE',  ( 1.000000000000000000, 0.000000000000000000, 0.000000000000000000 ) ) ;
#12745=ORIENTED_EDGE ( 'NONE', *, *, #15080, .T. ) ;
#12755=FACE_OUTER_BOUND ( 'NONE', #11782, .T. ) ;
#12775=CARTESIAN_POINT ( 'NONE',  ( 71.96535645333923981, 38.79159067395544014, 10.00000000000000178 ) ) ;
#12783=EDGE_CURVE ( 'NONE', #15168, #10673, #13498, .T. ) ;
#12786=CARTESIAN_POINT ( 'NONE',  ( -34.79899788034579444, 48.72489408690345414, 5.000000000000000000 ) ) ;
#12787=DIRECTION ( 'NONE',  ( -0.4873681696970814103, -0.8731965799097685110, -0.000000000000000000 ) ) ;
#12811=ADVANCED_FACE ( 'NONE', ( #1717 ), #5516, .T. ) ;
#12819=AXIS2_PLACEMENT_3D ( 'NONE', #7246, #1213, #100 ) ;
#12827=CARTESIAN_POINT ( 'NONE',  ( 169.5018791832601721, 101.0521538385604003, 5.000000000000000000 ) ) ;
#12842=AXIS2_PLACEMENT_3D ( 'NONE', #7272, #2602, #57 ) ;
#12847=AXIS2_PLACEMENT_3D ( 'NONE', #1037, #8247, #13023 ) ;
#12850=CIRCLE ( 'NONE', #12842, 5.000000000000004441 ) ;
#12856=DIRECTION ( 'NONE',  ( -0.000000000000000000, -0.000000000000000000, -1.000000000000000000 ) ) ;
#12864=VERTEX_POINT ( 'NONE', #7821 ) ;
#12885=AXIS2_PLACEMENT_3D ( 'NONE', #14750, #9728, #3948 ) ;
#12925=CYLINDRICAL_SURFACE ( 'NONE', #6002, 380.9270036976043343 ) ;
#12928=EDGE_CURVE ( 'NONE', #1071, #4381, #8138, .T. ) ;
#12931=ORIENTED_EDGE ( 'NONE', *, *, #13495, .T. ) ;
#12946=AXIS2_PLACEMENT_3D ( 'NONE', #2969, #11109, #7795 ) ;
#12949=ORIENTED_EDGE ( 'NONE', *, *, #3825, .T. ) ;
#12965=DIRECTION ( 'NONE',  ( 1.000000000000000000, 0.000000000000000000, 0.000000000000000000 ) ) ;
#12967=CARTESIAN_POINT ( 'NONE',  ( 170.2911098586863545, 111.9959133412127272, 0.000000000000000000 ) ) ;
#12975=AXIS2_PLACEMENT_3D ( 'NONE', #9578, #8329, #4520 ) ;
#12982=ADVANCED_FACE ( 'NONE', ( #6783 ), #14260, .F. ) ;
#12996=AXIS2_PLACEMENT_3D ( 'NONE', #5437, #15126, #11359 ) ;
#12997=DIRECTION ( 'NONE',  ( -0.000000000000000000, -0.000000000000000000, 1.000000000000000000 ) ) ;
#13003=CARTESIAN_POINT ( 'NONE',  ( -34.79899788034579444, 48.72489408690345414, 10.00000000000000178 ) ) ;
#13004=ORIENTED_EDGE ( 'NONE', *, *, #15132, .F. ) ;
#13006=DIRECTION ( 'NONE',  ( 0.000000000000000000, 0.000000000000000000, 1.000000000000000000 ) ) ;
#13019=EDGE_LOOP ( 'NONE', ( #13004, #2048 ) ) ;
#13021=CARTESIAN_POINT ( 'NONE',  ( -139.4318739252458670, 92.47118091487817537, 5.000000000000000000 ) ) ;
#13023=DIRECTION ( 'NONE',  ( 1.000000000000000000, 0.000000000000000000, 0.000000000000000000 ) ) ;
#13025=CARTESIAN_POINT ( 'NONE',  ( -156.6477983077465410, 110.1970436846185066, 0.000000000000000000 ) ) ;
#13026=ORIENTED_EDGE ( 'NONE', *, *, #11468, .T. ) ;
#13027=CARTESIAN_POINT ( 'NONE',  ( 122.5806775638430253, 45.00321902537314145, 5.000000000000000000 ) ) ;
#13061=CIRCLE ( 'NONE', #6276, 1.000000000000000888 ) ;
#13063=CARTESIAN_POINT ( 'NONE',  ( -130.9946291778373961, 96.97121815129470690, 5.000000000000000000 ) ) ;
#13071=DIRECTION ( 'NONE',  ( -1.000000000000000000, 0.000000000000000000, 0.000000000000000000 ) ) ;
#13073=CIRCLE ( 'NONE', #10323, 1.500000000000001332 ) ;
#13078=( NAMED_UNIT ( * ) PLANE_ANGLE_UNIT ( ) SI_UNIT ( $, .RADIAN. ) );
#13080=FACE_OUTER_BOUND ( 'NONE', #6241, .T. ) ;
#13084=CARTESIAN_POINT ( 'NONE',  ( 183.0404880503516267, 40.86394065090267702, 5.000000000000000000 ) ) ;
#13085=EDGE_CURVE ( 'NONE', #13090, #7984, #9953, .T. ) ;
#13089=AXIS2_PLACEMENT_3D ( 'NONE', #11320, #10453, #1992 ) ;
#13090=VERTEX_POINT ( 'NONE', #437 ) ;
#13113=VERTEX_POINT ( 'NONE', #6321 ) ;
#13122=VERTEX_POINT ( 'NONE', #1800 ) ;
#13132=CARTESIAN_POINT ( 'NONE',  ( 195.1062858801516597, 40.86394065090267702, 5.000000000000000000 ) ) ;
#13169=EDGE_LOOP ( 'NONE', ( #3065, #9665 ) ) ;
#13180=LINE ( 'NONE', #4663, #5588 ) ;
#13184=EDGE_CURVE ( 'NONE', #2617, #2533, #14697, .T. ) ;
#13188=FACE_OUTER_BOUND ( 'NONE', #14531, .T. ) ;
#13199=DIRECTION ( 'NONE',  ( 1.000000000000000000, 0.000000000000000000, 0.000000000000000000 ) ) ;
#13200=CARTESIAN_POINT ( 'NONE',  ( -150.4086188282879277, 107.2728346664360259, -5.000000000000000000 ) ) ;
#13249=LINE ( 'NONE', #2132, #7626 ) ;
#13254=DIRECTION ( 'NONE',  ( 1.000000000000000000, 0.000000000000000000, 0.000000000000000000 ) ) ;
#13256=ORIENTED_EDGE ( 'NONE', *, *, #839, .F. ) ;
#13261=ADVANCED_FACE ( 'NONE', ( #14028 ), #920, .F. ) ;
#13271=EDGE_LOOP ( 'NONE', ( #8677, #6226, #6976, #2234 ) ) ;
#13276=FACE_BOUND ( 'NONE', #6442, .T. ) ;
#13320=ADVANCED_FACE ( 'NONE', ( #6070 ), #2503, .F. ) ;
#13332=CARTESIAN_POINT ( 'NONE',  ( 174.2293059057019775, 61.25683321636181233, 0.000000000000000000 ) ) ;
#13346=FACE_OUTER_BOUND ( 'NONE', #6922, .T. ) ;
#13369=ORIENTED_EDGE ( 'NONE', *, *, #8208, .F. ) ;
#13391=ADVANCED_FACE ( 'NONE', ( #1312 ), #10963, .F. ) ;
#13397=VERTEX_POINT ( 'NONE', #3456 ) ;
#13406=AXIS2_PLACEMENT_3D ( 'NONE', #4565, #8225, #2274 ) ;
#13423=EDGE_LOOP ( 'NONE', ( #13026, #4298 ) ) ;
#13442=CARTESIAN_POINT ( 'NONE',  ( 200.1062858801516597, 40.86394065090267702, 0.000000000000000000 ) ) ;
#13466=PLANE ( 'NONE',  #7706 ) ;
#13470=ORIENTED_EDGE ( 'NONE', *, *, #10741, .F. ) ;
#13472=CIRCLE ( 'NONE', #860, 1.700000000000007061 ) ;
#13495=EDGE_CURVE ( 'NONE', #13816, #295, #4954, .T. ) ;
#13498=CIRCLE ( 'NONE', #12996, 10.97218105532926558 ) ;
#13504=CIRCLE ( 'NONE', #15268, 9.999999999999994671 ) ;
#13505=DIRECTION ( 'NONE',  ( -0.000000000000000000, -0.000000000000000000, -1.000000000000000000 ) ) ;
#13506=EDGE_LOOP ( 'NONE', ( #9148, #1336 ) ) ;
#13510=ORIENTED_EDGE ( 'NONE', *, *, #4068, .F. ) ;
#13511=EDGE_CURVE ( 'NONE', #295, #14046, #3377, .T. ) ;
#13525=ORIENTED_EDGE ( 'NONE', *, *, #11983, .T. ) ;
#13535=CARTESIAN_POINT ( 'NONE',  ( -136.9508382163321585, 108.2653706395415583, 0.000000000000000000 ) ) ;
#13582=AXIS2_PLACEMENT_3D ( 'NONE', #2478, #12033, #4931 ) ;
#13609=ORIENTED_EDGE ( 'NONE', *, *, #2366, .T. ) ;
#13615=DIRECTION ( 'NONE',  ( -0.000000000000000000, -0.000000000000000000, 1.000000000000000000 ) ) ;
#13636=AXIS2_PLACEMENT_3D ( 'NONE', #14210, #2140, #5704 ) ;
#13645=CIRCLE ( 'NONE', #1799, 1.700000000000007061 ) ;
#13651=VERTEX_POINT ( 'NONE', #13794 ) ;
#13697=VERTEX_POINT ( 'NONE', #6483 ) ;
#13728=LINE ( 'NONE', #14039, #1040 ) ;
#13741=DIRECTION ( 'NONE',  ( 1.000000000000000000, 0.000000000000000000, 0.000000000000000000 ) ) ;
#13742=ORIENTED_EDGE ( 'NONE', *, *, #10888, .T. ) ;
#13749=FACE_OUTER_BOUND ( 'NONE', #7135, .T. ) ;
#13752=ADVANCED_FACE ( 'NONE', ( #10413 ), #12925, .F. ) ;
#13781=CARTESIAN_POINT ( 'NONE',  ( -156.6477983077465410, 110.1970436846185066, -5.000000000000000000 ) ) ;
#13794=CARTESIAN_POINT ( 'NONE',  ( 15.71029453487719074, 40.04259805664093363, 5.000000000000000000 ) ) ;
#13798=VECTOR ( 'NONE', #14611, 1000.000000000000227 ) ;
#13802=CARTESIAN_POINT ( 'NONE',  ( -136.9508382163321585, 108.2653706395415441, 1.734723475976807094E-15 ) ) ;
#13816=VERTEX_POINT ( 'NONE', #4799 ) ;
#13822=ORIENTED_EDGE ( 'NONE', *, *, #3089, .F. ) ;
#13825=EDGE_CURVE ( 'NONE', #14046, #295, #11798, .T. ) ;
#13830=DIRECTION ( 'NONE',  ( -0.000000000000000000, -0.000000000000000000, 1.000000000000000000 ) ) ;
#13835=EDGE_CURVE ( 'NONE', #1269, #1785, #11500, .T. ) ;
#13839=ORIENTED_EDGE ( 'NONE', *, *, #401, .T. ) ;
#13840=DIRECTION ( 'NONE',  ( 0.8731965799097686221, -0.4873681696970814659, 0.000000000000000000 ) ) ;
#13843=DIRECTION ( 'NONE',  ( 0.000000000000000000, 0.000000000000000000, 1.000000000000000000 ) ) ;
#13862=EDGE_CURVE ( 'NONE', #14293, #873, #9576, .T. ) ;
#13868=ORIENTED_EDGE ( 'NONE', *, *, #13184, .T. ) ;
#13886=EDGE_LOOP ( 'NONE', ( #6373, #1270, #8663, #11123 ) ) ;
#13927=ORIENTED_EDGE ( 'NONE', *, *, #13511, .T. ) ;
#13944=PRODUCT ( 'Long Manual Lever Operating Handle', 'Long Manual Lever Operating Handle', '', ( #3092 ) ) ;
#13949=VERTEX_POINT ( 'NONE', #1742 ) ;
#13959=CARTESIAN_POINT ( 'NONE',  ( 19.11029453487719110, 40.04259805664093363, 10.00000000000000178 ) ) ;
#13976=( GEOMETRIC_REPRESENTATION_CONTEXT ( 3 ) GLOBAL_UNCERTAINTY_ASSIGNED_CONTEXT ( ( #11796 ) ) GLOBAL_UNIT_ASSIGNED_CONTEXT ( ( #4919, #3724, #307 ) ) REPRESENTATION_CONTEXT ( 'NONE', 'WORKASPACE' ) );
#13982=CARTESIAN_POINT ( 'NONE',  ( -164.5262273476079713, 106.7842295329138835, 5.000000000000000000 ) ) ;
#13985=DIRECTION ( 'NONE',  ( -0.000000000000000000, -0.000000000000000000, 1.000000000000000000 ) ) ;
#13988=VERTEX_POINT ( 'NONE', #545 ) ;
#13996=DIRECTION ( 'NONE',  ( 1.000000000000000000, 0.000000000000000000, 0.000000000000000000 ) ) ;
#14003=ORIENTED_EDGE ( 'NONE', *, *, #1163, .T. ) ;
#14017=CIRCLE ( 'NONE', #7992, 1.700000000000007061 ) ;
#14028=FACE_OUTER_BOUND ( 'NONE', #5765, .T. ) ;
#14039=CARTESIAN_POINT ( 'NONE',  ( -135.3034657297974093, 107.4444500778096483, 0.000000000000000000 ) ) ;
#14046=VERTEX_POINT ( 'NONE', #10725 ) ;
#14079=FACE_OUTER_BOUND ( 'NONE', #5194, .T. ) ;
#14107=DIRECTION ( 'NONE',  ( 0.000000000000000000, 0.000000000000000000, 1.000000000000000000 ) ) ;
#14114=DIRECTION ( 'NONE',  ( -0.000000000000000000, -0.000000000000000000, 1.000000000000000000 ) ) ;
#14119=CARTESIAN_POINT ( 'NONE',  ( -164.5262273476079713, 106.7842295329138835, 5.000000000000000000 ) ) ;
#14139=ORIENTED_EDGE ( 'NONE', *, *, #15238, .T. ) ;
#14142=CYLINDRICAL_SURFACE ( 'NONE', #8821, 17.06579782980005433 ) ;
#14147=DIRECTION ( 'NONE',  ( 0.000000000000000000, 0.000000000000000000, 1.000000000000000000 ) ) ;
#14160=CARTESIAN_POINT ( 'NONE',  ( -83.77455057502459113, 65.19100426474074084, 5.000000000000000000 ) ) ;
#14165=CIRCLE ( 'NONE', #8152, 54.67486482576605766 ) ;
#14168=DIRECTION ( 'NONE',  ( -0.000000000000000000, 0.000000000000000000, 1.000000000000000000 ) ) ;
#14174=DIRECTION ( 'NONE',  ( 1.000000000000000000, 0.000000000000000000, 0.000000000000000000 ) ) ;
#14186=DIRECTION ( 'NONE',  ( -0.8950274278067241740, 0.4460111024107797362, -0.000000000000000000 ) ) ;
#14188=DIRECTION ( 'NONE',  ( 1.000000000000000000, 0.000000000000000000, 0.000000000000000000 ) ) ;
#14209=DIRECTION ( 'NONE',  ( -0.000000000000000000, -0.000000000000000000, -1.000000000000000000 ) ) ;
#14210=CARTESIAN_POINT ( 'NONE',  ( 191.8042410000843745, 59.95507574834591225, 0.000000000000000000 ) ) ;
#14214=FACE_OUTER_BOUND ( 'NONE', #8700, .T. ) ;
#14216=DIRECTION ( 'NONE',  ( 0.000000000000000000, 0.000000000000000000, 1.000000000000000000 ) ) ;
#14226=DIRECTION ( 'NONE',  ( -0.000000000000000000, 0.000000000000000000, 1.000000000000000000 ) ) ;
#14253=DIRECTION ( 'NONE',  ( -0.000000000000000000, -0.000000000000000000, 1.000000000000000000 ) ) ;
#14254=DIRECTION ( 'NONE',  ( 1.000000000000000000, 0.000000000000000000, 0.000000000000000000 ) ) ;
#14260=CYLINDRICAL_SURFACE ( 'NONE', #3364, 1.000000000000000888 ) ;
#14269=CARTESIAN_POINT ( 'NONE',  ( 70.26535645333922275, 38.79159067395544014, 10.00000000000000178 ) ) ;
#14274=AXIS2_PLACEMENT_3D ( 'NONE', #3847, #1454, #12356 ) ;
#14280=VERTEX_POINT ( 'NONE', #2826 ) ;
#14288=CARTESIAN_POINT ( 'NONE',  ( 183.0404880503516267, 40.86394065090267702, 5.000000000000000000 ) ) ;
#14293=VERTEX_POINT ( 'NONE', #14728 ) ;
#14299=ORIENTED_EDGE ( 'NONE', *, *, #13085, .T. ) ;
#14325=CARTESIAN_POINT ( 'NONE',  ( -132.4907271922243694, 117.2156449176087847, 0.000000000000000000 ) ) ;
#14329=DIRECTION ( 'NONE',  ( -1.000000000000000000, 0.000000000000000000, 0.000000000000000000 ) ) ;
#14339=AXIS2_PLACEMENT_3D ( 'NONE', #5640, #14226, #11877 ) ;
#14345=DIRECTION ( 'NONE',  ( 1.000000000000000000, 0.000000000000000000, 0.000000000000000000 ) ) ;
#14362=AXIS2_PLACEMENT_3D ( 'NONE', #1681, #1835, #7539 ) ;
#14364=ORIENTED_EDGE ( 'NONE', *, *, #2457, .T. ) ;
#14392=ORIENTED_EDGE ( 'NONE', *, *, #5987, .F. ) ;
#14397=CARTESIAN_POINT ( 'NONE',  ( 200.1062858801516597, 40.86394065090267702, 5.000000000000000000 ) ) ;
#14408=LINE ( 'NONE', #15583, #9857 ) ;
#14469=STYLED_ITEM ( 'NONE', ( #7449 ), #11106 ) ;
#14481=ORIENTED_EDGE ( 'NONE', *, *, #6856, .F. ) ;
#14510=ORIENTED_EDGE ( 'NONE', *, *, #2967, .T. ) ;
#14511=ORIENTED_EDGE ( 'NONE', *, *, #10888, .F. ) ;
#14531=EDGE_LOOP ( 'NONE', ( #8317, #11489, #13839, #5725 ) ) ;
#14546=DIRECTION ( 'NONE',  ( -0.000000000000000000, -0.000000000000000000, 1.000000000000000000 ) ) ;
#14547=CARTESIAN_POINT ( 'NONE',  ( -132.4907271922243694, 117.2156449176087847, 5.000000000000000000 ) ) ;
#14564=DIRECTION ( 'NONE',  ( 0.000000000000000000, 0.000000000000000000, 1.000000000000000000 ) ) ;
#14565=DIRECTION ( 'NONE',  ( 0.000000000000000000, 0.000000000000000000, 1.000000000000000000 ) ) ;
#14587=EDGE_CURVE ( 'NONE', #6998, #7301, #2224, .T. ) ;
#14611=DIRECTION ( 'NONE',  ( -0.8950274278067241740, 0.4460111024107797362, -0.000000000000000000 ) ) ;
#14613=CARTESIAN_POINT ( 'NONE',  ( 190.2479883433758800, 63.36949047362622167, 0.000000000000000000 ) ) ;
#14614=DIRECTION ( 'NONE',  ( 1.000000000000000000, 0.000000000000000000, 0.000000000000000000 ) ) ;
#14625=EDGE_CURVE ( 'NONE', #13113, #14692, #10825, .T. ) ;
#14647=CLOSED_SHELL ( 'NONE', ( #1899, #8192, #535, #4500, #4474, #13320, #7625, #12275, #1523, #7701, #13752, #1648, #11631, #12152, #3525, #12529, #1059, #8656, #6694, #1694, #3917, #8816, #6320, #13261, #13391, #15613, #3240, #11136, #8567, #12032, #7193, #12811, #12982, #1201 ) ) ;
#14685=SURFACE_STYLE_USAGE ( .BOTH. , #14762 ) ;
#14692=VERTEX_POINT ( 'NONE', #3366 ) ;
#14697=CIRCLE ( 'NONE', #6904, 3.752352628381527833 ) ;
#14711=EDGE_CURVE ( 'NONE', #3245, #3263, #2498, .T. ) ;
#14728=CARTESIAN_POINT ( 'NONE',  ( -136.9508382163321585, 108.2653706395415583, 5.000000000000000000 ) ) ;
#14750=CARTESIAN_POINT ( 'NONE',  ( 13.07968152355895874, 460.3807876674321165, 0.000000000000000000 ) ) ;
#14762=SURFACE_SIDE_STYLE ('',( #9735 ) ) ;
#14769=EDGE_LOOP ( 'NONE', ( #15599, #6364, #13470, #3247 ) ) ;
#14791=LINE ( 'NONE', #12581, #5805 ) ;
#14792=EDGE_CURVE ( 'NONE', #14996, #2654, #26, .T. ) ;
#14797=DIRECTION ( 'NONE',  ( 0.000000000000000000, 0.000000000000000000, 1.000000000000000000 ) ) ;
#14822=DIRECTION ( 'NONE',  ( 0.000000000000000000, 0.000000000000000000, -1.000000000000000000 ) ) ;
#14841=EDGE_CURVE ( 'NONE', #9826, #1584, #3996, .T. ) ;
#14842=CARTESIAN_POINT ( 'NONE',  ( -85.27455057502459113, 65.19100426474074084, 0.000000000000000000 ) ) ;
#14857=AXIS2_PLACEMENT_3D ( 'NONE', #11395, #7620, #1598 ) ;
#14881=FACE_OUTER_BOUND ( 'NONE', #10589, .T. ) ;
#14886=EDGE_LOOP ( 'NONE', ( #10811, #12931, #13927, #8230 ) ) ;
#14897=VECTOR ( 'NONE', #6889, 1000.000000000000000 ) ;
#14905=ORIENTED_EDGE ( 'NONE', *, *, #822, .F. ) ;
#14925=ORIENTED_EDGE ( 'NONE', *, *, #1508, .F. ) ;
#14946=VECTOR ( 'NONE', #4161, 1000.000000000000227 ) ;
#14964=AXIS2_PLACEMENT_3D ( 'NONE', #10925, #2547, #4993 ) ;
#14981=VERTEX_POINT ( 'NONE', #4206 ) ;
#14989=EDGE_CURVE ( 'NONE', #13397, #11374, #13061, .T. ) ;
#14996=VERTEX_POINT ( 'NONE', #12423 ) ;
#15012=EDGE_CURVE ( 'NONE', #5538, #13816, #8309, .T. ) ;
#15049=FACE_BOUND ( 'NONE', #2356, .T. ) ;
#15080=EDGE_CURVE ( 'NONE', #12631, #462, #3769, .T. ) ;
#15100=EDGE_CURVE ( 'NONE', #5874, #555, #15482, .T. ) ;
#15116=EDGE_LOOP ( 'NONE', ( #4739, #955, #12075, #13609 ) ) ;
#15117=EDGE_LOOP ( 'NONE', ( #14299, #6663, #8118, #10003 ) ) ;
#15120=CARTESIAN_POINT ( 'NONE',  ( 193.3006371371548369, 56.51400776751751920, 5.000000000000000000 ) ) ;
#15126=DIRECTION ( 'NONE',  ( 0.000000000000000000, 0.000000000000000000, 1.000000000000000000 ) ) ;
#15132=EDGE_CURVE ( 'NONE', #11374, #13397, #5535, .T. ) ;
#15133=CARTESIAN_POINT ( 'NONE',  ( 13.07968152355895874, 460.3807876674321165, 5.000000000000000000 ) ) ;
#15137=CARTESIAN_POINT ( 'NONE',  ( 174.2293059057019775, 61.25683321636181233, 10.00000000000000178 ) ) ;
#15144=DIRECTION ( 'NONE',  ( 0.000000000000000000, 0.000000000000000000, 1.000000000000000000 ) ) ;
#15157=CARTESIAN_POINT ( 'NONE',  ( -36.49899788034579018, 48.72489408690345414, 10.00000000000000178 ) ) ;
#15168=VERTEX_POINT ( 'NONE', #12967 ) ;
#15178=FACE_BOUND ( 'NONE', #230, .T. ) ;
#15186=AXIS2_PLACEMENT_3D ( 'NONE', #5458, #12630, #6802 ) ;
#15187=EDGE_LOOP ( 'NONE', ( #10601, #8313, #11804, #7195 ) ) ;
#15199=LINE ( 'NONE', #15120, #12049 ) ;
#15208=CARTESIAN_POINT ( 'NONE',  ( 191.8042410000843745, 59.95507574834591225, 5.000000000000000000 ) ) ;
#15238=EDGE_CURVE ( 'NONE', #2617, #12412, #9663, .T. ) ;
#15261=CARTESIAN_POINT ( 'NONE',  ( -157.8787660911425803, 118.6941998492684149, 5.000000000000000000 ) ) ;
#15268=AXIS2_PLACEMENT_3D ( 'NONE', #13063, #10007, #7560 ) ;
#15278=DIRECTION ( 'NONE',  ( 1.000000000000000000, 0.000000000000000000, 0.000000000000000000 ) ) ;
#15283=EDGE_LOOP ( 'NONE', ( #12676, #2999 ) ) ;
#15284=( LENGTH_UNIT ( ) NAMED_UNIT ( * ) SI_UNIT ( .MILLI., .METRE. ) );
#15293=EDGE_CURVE ( 'NONE', #3314, #4062, #4252, .T. ) ;
#15303=APPLICATION_CONTEXT ( 'automotive_design' ) ;
#15307=CARTESIAN_POINT ( 'NONE',  ( -144.0627431139473345, 95.36268816863731956, 5.000000000000000000 ) ) ;
#15320=ORIENTED_EDGE ( 'NONE', *, *, #7394, .F. ) ;
#15360=EDGE_CURVE ( 'NONE', #2732, #14981, #11831, .T. ) ;
#15400=AXIS2_PLACEMENT_3D ( 'NONE', #14397, #9915, #11017 ) ;
#15451=EDGE_CURVE ( 'NONE', #1469, #13988, #13073, .T. ) ;
#15457=AXIS2_PLACEMENT_3D ( 'NONE', #344, #14564, #5183 ) ;
#15465=ORIENTED_EDGE ( 'NONE', *, *, #9364, .F. ) ;
#15476=EDGE_CURVE ( 'NONE', #873, #4947, #5623, .T. ) ;
#15482=LINE ( 'NONE', #3497, #7312 ) ;
#15489=DIRECTION ( 'NONE',  ( 0.000000000000000000, 0.000000000000000000, 1.000000000000000000 ) ) ;
#15492=AXIS2_PLACEMENT_3D ( 'NONE', #4204, #13840, #1839 ) ;
#15516=CIRCLE ( 'NONE', #9000, 17.06579782980005433 ) ;
#15577=ORIENTED_EDGE ( 'NONE', *, *, #13835, .F. ) ;
#15583=CARTESIAN_POINT ( 'NONE',  ( -33.09899788034579871, 48.72489408690345414, 10.00000000000000178 ) ) ;
#15584=FACE_OUTER_BOUND ( 'NONE', #6031, .T. ) ;
#15588=CARTESIAN_POINT ( 'NONE',  ( 200.1062858801516597, 40.86394065090267702, 5.000000000000000000 ) ) ;
#15599=ORIENTED_EDGE ( 'NONE', *, *, #11356, .T. ) ;
#15609=LINE ( 'NONE', #8460, #3531 ) ;
#15613=ADVANCED_FACE ( 'NONE', ( #11605 ), #768, .F. ) ;
ENDSEC;
END-ISO-10303-21;
